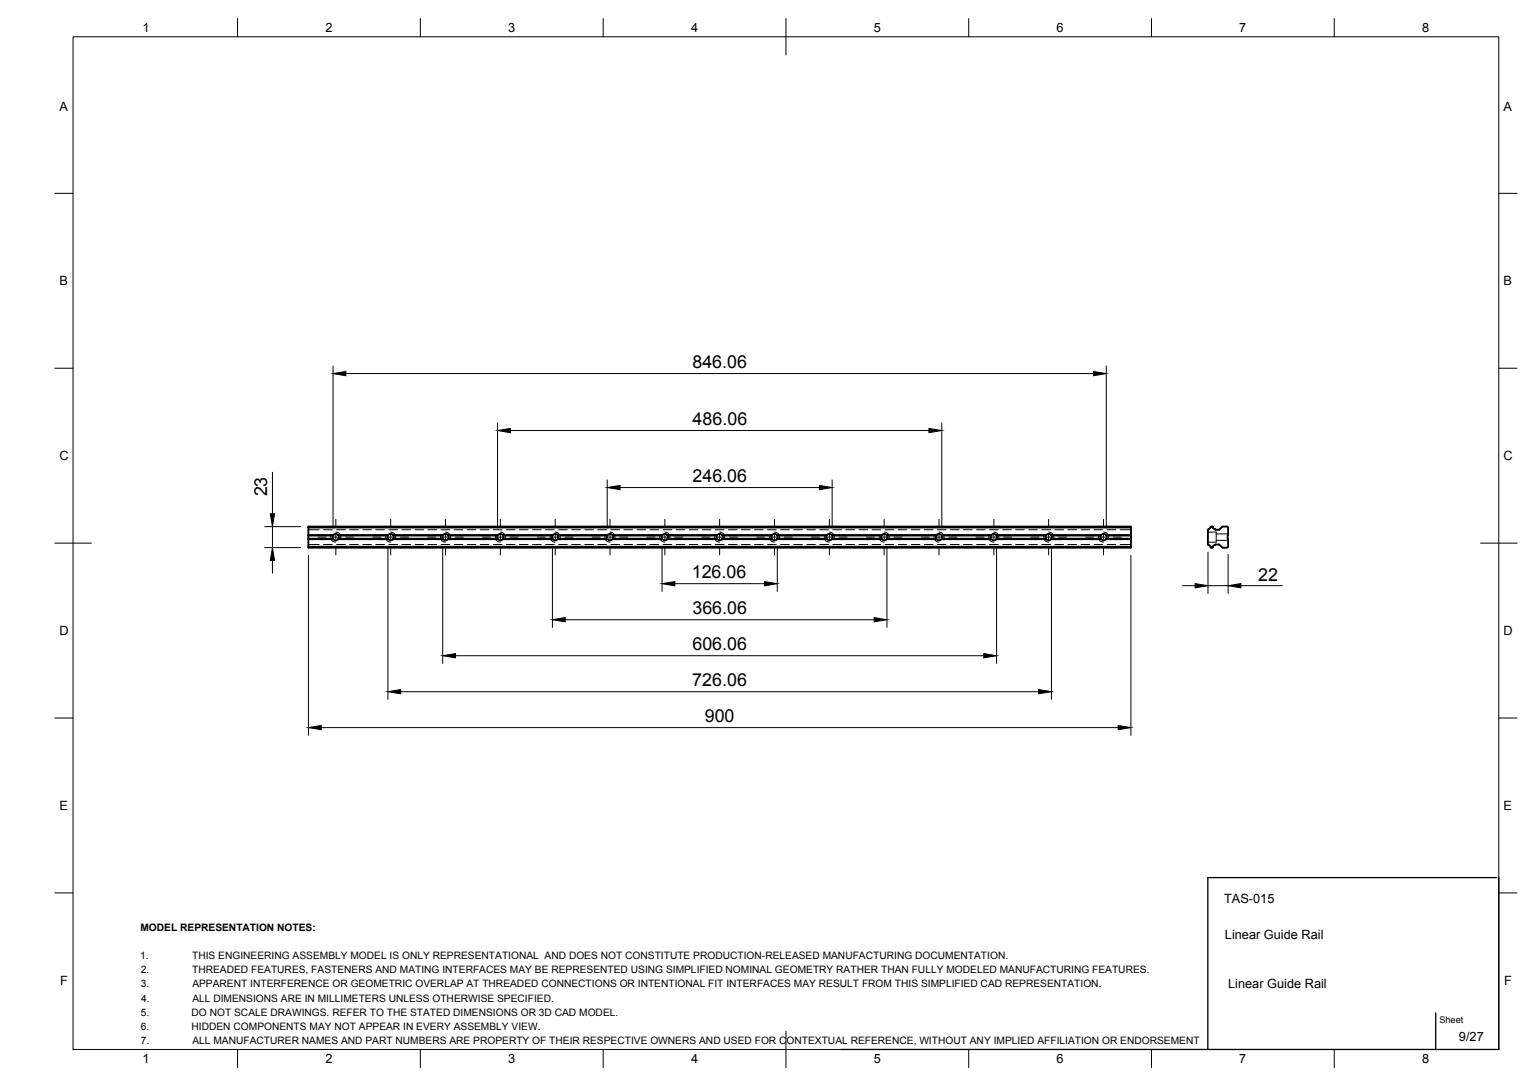
ISO-10303-21;
HEADER;
/* Generated by software containing ST-Developer
 * from STEP Tools, Inc. (www.steptools.com) 
 */

FILE_DESCRIPTION(
/* description */ ('STEP AP214'),
/* implementation_level */ '2;1');

FILE_NAME(
/* name */ 'Linear Guide Rail.step',
/* time_stamp */ '2026-11-15T14:49:54-08:00',
/* author */ (''),
/* organization */ (''),
/* preprocessor_version */ 'ST-DEVELOPER v20.2',
/* originating_system */ 'Autodesk Translation Framework v15.17.0.0',
/* authorisation */ '');

FILE_SCHEMA (('AUTOMOTIVE_DESIGN { 1 0 10303 214 3 1 1 }'));
ENDSEC;

DATA;
#10=MECHANICAL_DESIGN_GEOMETRIC_PRESENTATION_REPRESENTATION('',(#1104),#66721);
#582=ELLIPSE('',#26235,4.94974735819038,3.49999990182558);
#583=ELLIPSE('',#26237,4.94974766602105,3.5000001764392);
#584=ELLIPSE('',#26241,4.94974746762207,3.49999999945822);
#585=ELLIPSE('',#26243,4.94974743837769,3.49999997319395);
#586=ELLIPSE('',#26249,4.94974746471116,3.49999999781732);
#587=ELLIPSE('',#26251,4.94974761521235,3.50000013143823);
#588=ELLIPSE('',#26255,4.94974751536128,3.5000000426592);
#589=ELLIPSE('',#26257,4.94974734791332,3.49999989298097);
#590=ELLIPSE('',#26263,4.94974738455087,3.49999992654364);
#591=ELLIPSE('',#26265,4.94974756609828,3.50000008750549);
#592=ELLIPSE('',#26269,4.94974748465299,3.50000001559145);
#593=ELLIPSE('',#26271,4.9497474078675,3.49999994629514);
#594=ELLIPSE('',#26277,4.9497473461591,3.49999989191482);
#595=ELLIPSE('',#26279,4.94974750610666,3.50000003412937);
#596=ELLIPSE('',#26283,4.94974748783974,3.50000001743086);
#597=ELLIPSE('',#26285,4.94974744634947,3.49999998103439);
#598=ELLIPSE('',#26291,4.94974749695506,3.50000002579411);
#599=ELLIPSE('',#26293,4.94974750752024,3.50000003493957);
#600=ELLIPSE('',#26297,4.94974751315491,3.50000003982775);
#601=ELLIPSE('',#26299,4.949747463355,3.4999999955299);
#602=ELLIPSE('',#26305,4.94974749836308,3.50000002653739);
#603=ELLIPSE('',#26307,4.94974757675016,3.50000009672614);
#604=ELLIPSE('',#26311,4.94974748001691,3.50000000973653);
#605=ELLIPSE('',#26313,4.94974739716868,3.49999993702713);
#606=ELLIPSE('',#26319,4.94974749924226,3.5000000270794);
#607=ELLIPSE('',#26321,4.94974743684973,3.49999997233704);
#608=ELLIPSE('',#26325,4.9497475382208,3.50000006223073);
#609=ELLIPSE('',#26327,4.94974747235583,3.5000000037591);
#610=ELLIPSE('',#26333,4.94974748843076,3.5000000176963);
#611=ELLIPSE('',#26335,4.94974741762146,3.49999995499458);
#612=ELLIPSE('',#26339,4.94974749231943,3.50000002155544);
#613=ELLIPSE('',#26341,4.94974745849775,3.49999999105758);
#614=ELLIPSE('',#26347,4.94974743835813,3.49999997320228);
#615=ELLIPSE('',#26349,4.94974746762365,3.49999999944211);
#616=ELLIPSE('',#26353,4.94974749229401,3.50000002151707);
#617=ELLIPSE('',#26355,4.9497474430954,3.4999999775075);
#618=ELLIPSE('',#26361,4.94974746457826,3.49999999694589);
#619=ELLIPSE('',#26363,4.94974746001076,3.49999999272877);
#620=ELLIPSE('',#26367,4.94974748578252,3.50000001541321);
#621=ELLIPSE('',#26369,4.94974746533883,3.49999999735002);
#622=ELLIPSE('',#26375,4.94974749254742,3.50000002161139);
#623=ELLIPSE('',#26377,4.94974746567926,3.49999999752504);
#624=ELLIPSE('',#26381,4.94974748072687,3.50000001091353);
#625=ELLIPSE('',#26383,4.94974746232603,3.49999999483898);
#626=ELLIPSE('',#26389,4.94974748208041,3.50000001242701);
#627=ELLIPSE('',#26391,4.94974745070612,3.49999998421949);
#628=ELLIPSE('',#26395,4.94974745801903,3.49999999076925);
#629=ELLIPSE('',#26397,4.94974746302533,3.49999999523587);
#630=ELLIPSE('',#26403,4.94974746046047,3.49999999301059);
#631=ELLIPSE('',#26405,4.94974745907472,3.49999999180994);
#632=ELLIPSE('',#26409,4.94974747036828,3.50000000182558);
#633=ELLIPSE('',#26411,4.9497474701889,3.50000000171811);
#634=ELLIPSE('',#26417,4.94974746606674,3.49999999798426);
#635=ELLIPSE('',#26419,4.94974746678755,3.49999999861078);
#636=ELLIPSE('',#26423,4.94974746786117,3.49999999962962);
#637=ELLIPSE('',#26425,4.9497474685907,3.50000000019107);
#638=ELLIPSE('',#26431,4.94974746853076,3.50000000020001);
#639=ELLIPSE('',#26433,4.94974746847046,3.50000000014575);
#640=ELLIPSE('',#26437,4.9497474687332,3.50000000037123);
#641=ELLIPSE('',#26439,4.94974746865778,3.50000000030521);
#1042=SHAPE_REPRESENTATION_RELATIONSHIP('SRR','None',#66900,#1073);
#1073=ADVANCED_BREP_SHAPE_REPRESENTATION('',(#1139),#66691);
#1104=STYLED_ITEM('',(#67095),#1139);
#1139=MANIFOLD_SOLID_BREP('Body1',#25670);
#1247=FACE_BOUND('',#3970,.T.);
#1248=FACE_BOUND('',#3971,.T.);
#1249=FACE_BOUND('',#3972,.T.);
#1250=FACE_BOUND('',#3973,.T.);
#1251=FACE_BOUND('',#3974,.T.);
#1252=FACE_BOUND('',#3975,.T.);
#1253=FACE_BOUND('',#3976,.T.);
#1254=FACE_BOUND('',#3977,.T.);
#1255=FACE_BOUND('',#3978,.T.);
#1256=FACE_BOUND('',#3979,.T.);
#1257=FACE_BOUND('',#3980,.T.);
#1258=FACE_BOUND('',#3981,.T.);
#1259=FACE_BOUND('',#3982,.T.);
#1260=FACE_BOUND('',#3983,.T.);
#1261=FACE_BOUND('',#3984,.T.);
#1262=FACE_BOUND('',#4023,.T.);
#1263=FACE_BOUND('',#4025,.T.);
#1264=FACE_BOUND('',#4027,.T.);
#1265=FACE_BOUND('',#4029,.T.);
#1266=FACE_BOUND('',#4031,.T.);
#1267=FACE_BOUND('',#4033,.T.);
#1268=FACE_BOUND('',#4035,.T.);
#1269=FACE_BOUND('',#4037,.T.);
#1270=FACE_BOUND('',#4039,.T.);
#1271=FACE_BOUND('',#4041,.T.);
#1272=FACE_BOUND('',#4043,.T.);
#1273=FACE_BOUND('',#4045,.T.);
#1274=FACE_BOUND('',#4047,.T.);
#1275=FACE_BOUND('',#4049,.T.);
#1276=FACE_BOUND('',#4051,.T.);
#1551=PLANE('',#26440);
#1552=PLANE('',#26441);
#1553=PLANE('',#26442);
#1554=PLANE('',#26443);
#1555=PLANE('',#26444);
#1556=PLANE('',#26445);
#1557=PLANE('',#26446);
#1558=PLANE('',#26447);
#1559=PLANE('',#26448);
#1560=PLANE('',#26449);
#1561=PLANE('',#26450);
#1562=PLANE('',#26451);
#1563=PLANE('',#26452);
#1564=PLANE('',#26453);
#1565=PLANE('',#26454);
#1566=PLANE('',#26455);
#1567=PLANE('',#26456);
#1568=PLANE('',#26457);
#1569=PLANE('',#26458);
#1570=PLANE('',#26459);
#1571=PLANE('',#26460);
#1572=PLANE('',#26461);
#1573=PLANE('',#26462);
#1574=PLANE('',#26463);
#1575=PLANE('',#26464);
#1576=PLANE('',#26465);
#1577=PLANE('',#26466);
#1578=PLANE('',#26467);
#1579=PLANE('',#26468);
#1580=PLANE('',#26469);
#1581=PLANE('',#26470);
#1582=PLANE('',#26471);
#1583=PLANE('',#26472);
#1584=PLANE('',#26473);
#1585=PLANE('',#26474);
#1586=PLANE('',#26475);
#1587=PLANE('',#26476);
#1588=PLANE('',#26477);
#1589=PLANE('',#26478);
#1590=PLANE('',#26479);
#1591=PLANE('',#26480);
#1592=PLANE('',#26481);
#1593=PLANE('',#26482);
#1594=PLANE('',#26483);
#1595=PLANE('',#26484);
#1596=PLANE('',#26485);
#1597=PLANE('',#26486);
#1598=PLANE('',#26487);
#1599=PLANE('',#26510);
#1600=PLANE('',#26533);
#1601=PLANE('',#26534);
#1602=PLANE('',#26535);
#1603=PLANE('',#26536);
#1604=PLANE('',#26537);
#1605=PLANE('',#26538);
#1606=PLANE('',#26539);
#1607=PLANE('',#26540);
#1608=PLANE('',#26541);
#1609=PLANE('',#26542);
#1610=PLANE('',#26543);
#1611=PLANE('',#26544);
#1612=PLANE('',#26545);
#1613=PLANE('',#26546);
#1614=PLANE('',#26558);
#1615=PLANE('',#26559);
#1616=PLANE('',#26560);
#1617=PLANE('',#26561);
#1618=PLANE('',#26562);
#1619=PLANE('',#26574);
#1620=PLANE('',#26575);
#1621=PLANE('',#26576);
#1622=PLANE('',#26577);
#1623=PLANE('',#26578);
#1624=PLANE('',#26579);
#1625=PLANE('',#26580);
#1626=PLANE('',#26581);
#1627=PLANE('',#26582);
#1628=PLANE('',#26583);
#1629=PLANE('',#26584);
#1630=PLANE('',#26585);
#1631=PLANE('',#26586);
#1632=PLANE('',#26587);
#1633=PLANE('',#26588);
#1634=PLANE('',#26589);
#1635=PLANE('',#26590);
#1636=PLANE('',#26591);
#2363=FACE_OUTER_BOUND('',#3884,.T.);
#2364=FACE_OUTER_BOUND('',#3885,.T.);
#2365=FACE_OUTER_BOUND('',#3886,.T.);
#2366=FACE_OUTER_BOUND('',#3887,.T.);
#2367=FACE_OUTER_BOUND('',#3888,.T.);
#2368=FACE_OUTER_BOUND('',#3889,.T.);
#2369=FACE_OUTER_BOUND('',#3890,.T.);
#2370=FACE_OUTER_BOUND('',#3891,.T.);
#2371=FACE_OUTER_BOUND('',#3892,.T.);
#2372=FACE_OUTER_BOUND('',#3893,.T.);
#2373=FACE_OUTER_BOUND('',#3894,.T.);
#2374=FACE_OUTER_BOUND('',#3895,.T.);
#2375=FACE_OUTER_BOUND('',#3896,.T.);
#2376=FACE_OUTER_BOUND('',#3897,.T.);
#2377=FACE_OUTER_BOUND('',#3898,.T.);
#2378=FACE_OUTER_BOUND('',#3899,.T.);
#2379=FACE_OUTER_BOUND('',#3900,.T.);
#2380=FACE_OUTER_BOUND('',#3901,.T.);
#2381=FACE_OUTER_BOUND('',#3902,.T.);
#2382=FACE_OUTER_BOUND('',#3903,.T.);
#2383=FACE_OUTER_BOUND('',#3904,.T.);
#2384=FACE_OUTER_BOUND('',#3905,.T.);
#2385=FACE_OUTER_BOUND('',#3906,.T.);
#2386=FACE_OUTER_BOUND('',#3907,.T.);
#2387=FACE_OUTER_BOUND('',#3908,.T.);
#2388=FACE_OUTER_BOUND('',#3909,.T.);
#2389=FACE_OUTER_BOUND('',#3910,.T.);
#2390=FACE_OUTER_BOUND('',#3911,.T.);
#2391=FACE_OUTER_BOUND('',#3912,.T.);
#2392=FACE_OUTER_BOUND('',#3913,.T.);
#2393=FACE_OUTER_BOUND('',#3914,.T.);
#2394=FACE_OUTER_BOUND('',#3915,.T.);
#2395=FACE_OUTER_BOUND('',#3916,.T.);
#2396=FACE_OUTER_BOUND('',#3917,.T.);
#2397=FACE_OUTER_BOUND('',#3918,.T.);
#2398=FACE_OUTER_BOUND('',#3919,.T.);
#2399=FACE_OUTER_BOUND('',#3920,.T.);
#2400=FACE_OUTER_BOUND('',#3921,.T.);
#2401=FACE_OUTER_BOUND('',#3922,.T.);
#2402=FACE_OUTER_BOUND('',#3923,.T.);
#2403=FACE_OUTER_BOUND('',#3924,.T.);
#2404=FACE_OUTER_BOUND('',#3925,.T.);
#2405=FACE_OUTER_BOUND('',#3926,.T.);
#2406=FACE_OUTER_BOUND('',#3927,.T.);
#2407=FACE_OUTER_BOUND('',#3928,.T.);
#2408=FACE_OUTER_BOUND('',#3929,.T.);
#2409=FACE_OUTER_BOUND('',#3930,.T.);
#2410=FACE_OUTER_BOUND('',#3931,.T.);
#2411=FACE_OUTER_BOUND('',#3932,.T.);
#2412=FACE_OUTER_BOUND('',#3933,.T.);
#2413=FACE_OUTER_BOUND('',#3934,.T.);
#2414=FACE_OUTER_BOUND('',#3935,.T.);
#2415=FACE_OUTER_BOUND('',#3936,.T.);
#2416=FACE_OUTER_BOUND('',#3937,.T.);
#2417=FACE_OUTER_BOUND('',#3938,.T.);
#2418=FACE_OUTER_BOUND('',#3939,.T.);
#2419=FACE_OUTER_BOUND('',#3940,.T.);
#2420=FACE_OUTER_BOUND('',#3941,.T.);
#2421=FACE_OUTER_BOUND('',#3942,.T.);
#2422=FACE_OUTER_BOUND('',#3943,.T.);
#2423=FACE_OUTER_BOUND('',#3944,.T.);
#2424=FACE_OUTER_BOUND('',#3945,.T.);
#2425=FACE_OUTER_BOUND('',#3946,.T.);
#2426=FACE_OUTER_BOUND('',#3947,.T.);
#2427=FACE_OUTER_BOUND('',#3948,.T.);
#2428=FACE_OUTER_BOUND('',#3949,.T.);
#2429=FACE_OUTER_BOUND('',#3950,.T.);
#2430=FACE_OUTER_BOUND('',#3951,.T.);
#2431=FACE_OUTER_BOUND('',#3952,.T.);
#2432=FACE_OUTER_BOUND('',#3953,.T.);
#2433=FACE_OUTER_BOUND('',#3954,.T.);
#2434=FACE_OUTER_BOUND('',#3955,.T.);
#2435=FACE_OUTER_BOUND('',#3956,.T.);
#2436=FACE_OUTER_BOUND('',#3957,.T.);
#2437=FACE_OUTER_BOUND('',#3958,.T.);
#2438=FACE_OUTER_BOUND('',#3959,.T.);
#2439=FACE_OUTER_BOUND('',#3960,.T.);
#2440=FACE_OUTER_BOUND('',#3961,.T.);
#2441=FACE_OUTER_BOUND('',#3962,.T.);
#2442=FACE_OUTER_BOUND('',#3963,.T.);
#2443=FACE_OUTER_BOUND('',#3964,.T.);
#2444=FACE_OUTER_BOUND('',#3965,.T.);
#2445=FACE_OUTER_BOUND('',#3966,.T.);
#2446=FACE_OUTER_BOUND('',#3967,.T.);
#2447=FACE_OUTER_BOUND('',#3968,.T.);
#2448=FACE_OUTER_BOUND('',#3969,.T.);
#2449=FACE_OUTER_BOUND('',#3985,.T.);
#2450=FACE_OUTER_BOUND('',#3986,.T.);
#2451=FACE_OUTER_BOUND('',#3987,.T.);
#2452=FACE_OUTER_BOUND('',#3988,.T.);
#2453=FACE_OUTER_BOUND('',#3989,.T.);
#2454=FACE_OUTER_BOUND('',#3990,.T.);
#2455=FACE_OUTER_BOUND('',#3991,.T.);
#2456=FACE_OUTER_BOUND('',#3992,.T.);
#2457=FACE_OUTER_BOUND('',#3993,.T.);
#2458=FACE_OUTER_BOUND('',#3994,.T.);
#2459=FACE_OUTER_BOUND('',#3995,.T.);
#2460=FACE_OUTER_BOUND('',#3996,.T.);
#2461=FACE_OUTER_BOUND('',#3997,.T.);
#2462=FACE_OUTER_BOUND('',#3998,.T.);
#2463=FACE_OUTER_BOUND('',#3999,.T.);
#2464=FACE_OUTER_BOUND('',#4000,.T.);
#2465=FACE_OUTER_BOUND('',#4001,.T.);
#2466=FACE_OUTER_BOUND('',#4002,.T.);
#2467=FACE_OUTER_BOUND('',#4003,.T.);
#2468=FACE_OUTER_BOUND('',#4004,.T.);
#2469=FACE_OUTER_BOUND('',#4005,.T.);
#2470=FACE_OUTER_BOUND('',#4006,.T.);
#2471=FACE_OUTER_BOUND('',#4007,.T.);
#2472=FACE_OUTER_BOUND('',#4008,.T.);
#2473=FACE_OUTER_BOUND('',#4009,.T.);
#2474=FACE_OUTER_BOUND('',#4010,.T.);
#2475=FACE_OUTER_BOUND('',#4011,.T.);
#2476=FACE_OUTER_BOUND('',#4012,.T.);
#2477=FACE_OUTER_BOUND('',#4013,.T.);
#2478=FACE_OUTER_BOUND('',#4014,.T.);
#2479=FACE_OUTER_BOUND('',#4015,.T.);
#2480=FACE_OUTER_BOUND('',#4016,.T.);
#2481=FACE_OUTER_BOUND('',#4017,.T.);
#2482=FACE_OUTER_BOUND('',#4018,.T.);
#2483=FACE_OUTER_BOUND('',#4019,.T.);
#2484=FACE_OUTER_BOUND('',#4020,.T.);
#2485=FACE_OUTER_BOUND('',#4021,.T.);
#2486=FACE_OUTER_BOUND('',#4022,.T.);
#2487=FACE_OUTER_BOUND('',#4024,.T.);
#2488=FACE_OUTER_BOUND('',#4026,.T.);
#2489=FACE_OUTER_BOUND('',#4028,.T.);
#2490=FACE_OUTER_BOUND('',#4030,.T.);
#2491=FACE_OUTER_BOUND('',#4032,.T.);
#2492=FACE_OUTER_BOUND('',#4034,.T.);
#2493=FACE_OUTER_BOUND('',#4036,.T.);
#2494=FACE_OUTER_BOUND('',#4038,.T.);
#2495=FACE_OUTER_BOUND('',#4040,.T.);
#2496=FACE_OUTER_BOUND('',#4042,.T.);
#2497=FACE_OUTER_BOUND('',#4044,.T.);
#2498=FACE_OUTER_BOUND('',#4046,.T.);
#2499=FACE_OUTER_BOUND('',#4048,.T.);
#2500=FACE_OUTER_BOUND('',#4050,.T.);
#3884=EDGE_LOOP('',(#17068,#17069,#17070,#17071));
#3885=EDGE_LOOP('',(#17072,#17073,#17074,#17075,#17076,#17077,#17078,#17079,
#17080,#17081,#17082,#17083));
#3886=EDGE_LOOP('',(#17084,#17085,#17086,#17087));
#3887=EDGE_LOOP('',(#17088,#17089,#17090,#17091,#17092,#17093,#17094,#17095,
#17096,#17097,#17098,#17099));
#3888=EDGE_LOOP('',(#17100,#17101,#17102,#17103));
#3889=EDGE_LOOP('',(#17104,#17105,#17106,#17107,#17108,#17109,#17110,#17111,
#17112,#17113,#17114,#17115));
#3890=EDGE_LOOP('',(#17116,#17117,#17118,#17119));
#3891=EDGE_LOOP('',(#17120,#17121,#17122,#17123,#17124,#17125,#17126,#17127,
#17128,#17129,#17130,#17131));
#3892=EDGE_LOOP('',(#17132,#17133,#17134,#17135));
#3893=EDGE_LOOP('',(#17136,#17137,#17138,#17139,#17140,#17141,#17142,#17143,
#17144,#17145,#17146,#17147));
#3894=EDGE_LOOP('',(#17148,#17149,#17150,#17151));
#3895=EDGE_LOOP('',(#17152,#17153,#17154,#17155,#17156,#17157,#17158,#17159,
#17160,#17161,#17162,#17163));
#3896=EDGE_LOOP('',(#17164,#17165,#17166,#17167));
#3897=EDGE_LOOP('',(#17168,#17169,#17170,#17171,#17172,#17173,#17174,#17175,
#17176,#17177,#17178,#17179));
#3898=EDGE_LOOP('',(#17180,#17181,#17182,#17183));
#3899=EDGE_LOOP('',(#17184,#17185,#17186,#17187,#17188,#17189,#17190,#17191,
#17192,#17193,#17194,#17195));
#3900=EDGE_LOOP('',(#17196,#17197,#17198,#17199));
#3901=EDGE_LOOP('',(#17200,#17201,#17202,#17203,#17204,#17205,#17206,#17207,
#17208,#17209,#17210,#17211));
#3902=EDGE_LOOP('',(#17212,#17213,#17214,#17215));
#3903=EDGE_LOOP('',(#17216,#17217,#17218,#17219,#17220,#17221,#17222,#17223,
#17224,#17225,#17226,#17227));
#3904=EDGE_LOOP('',(#17228,#17229,#17230,#17231));
#3905=EDGE_LOOP('',(#17232,#17233,#17234,#17235,#17236,#17237,#17238,#17239,
#17240,#17241,#17242,#17243));
#3906=EDGE_LOOP('',(#17244,#17245,#17246,#17247));
#3907=EDGE_LOOP('',(#17248,#17249,#17250,#17251,#17252,#17253,#17254,#17255,
#17256,#17257,#17258,#17259));
#3908=EDGE_LOOP('',(#17260,#17261,#17262,#17263));
#3909=EDGE_LOOP('',(#17264,#17265,#17266,#17267,#17268,#17269,#17270,#17271,
#17272,#17273,#17274,#17275));
#3910=EDGE_LOOP('',(#17276,#17277,#17278,#17279));
#3911=EDGE_LOOP('',(#17280,#17281,#17282,#17283,#17284,#17285,#17286,#17287,
#17288,#17289,#17290,#17291));
#3912=EDGE_LOOP('',(#17292,#17293,#17294,#17295));
#3913=EDGE_LOOP('',(#17296,#17297,#17298,#17299,#17300,#17301,#17302,#17303,
#17304,#17305,#17306,#17307));
#3914=EDGE_LOOP('',(#17308,#17309,#17310,#17311));
#3915=EDGE_LOOP('',(#17312,#17313,#17314,#17315));
#3916=EDGE_LOOP('',(#17316,#17317,#17318,#17319,#17320,#17321,#17322,#17323,
#17324,#17325,#17326,#17327,#17328,#17329,#17330,#17331,#17332,#17333,#17334,
#17335,#17336,#17337,#17338,#17339,#17340,#17341,#17342,#17343,#17344,#17345,
#17346,#17347,#17348,#17349));
#3917=EDGE_LOOP('',(#17350,#17351,#17352,#17353,#17354));
#3918=EDGE_LOOP('',(#17355,#17356,#17357,#17358,#17359,#17360,#17361,#17362,
#17363,#17364,#17365,#17366,#17367,#17368,#17369,#17370,#17371,#17372,#17373,
#17374,#17375,#17376,#17377,#17378,#17379,#17380,#17381,#17382,#17383,#17384,
#17385,#17386,#17387,#17388));
#3919=EDGE_LOOP('',(#17389,#17390,#17391,#17392));
#3920=EDGE_LOOP('',(#17393,#17394,#17395,#17396,#17397));
#3921=EDGE_LOOP('',(#17398,#17399,#17400,#17401));
#3922=EDGE_LOOP('',(#17402,#17403,#17404,#17405));
#3923=EDGE_LOOP('',(#17406,#17407,#17408,#17409,#17410));
#3924=EDGE_LOOP('',(#17411,#17412,#17413,#17414));
#3925=EDGE_LOOP('',(#17415,#17416,#17417,#17418));
#3926=EDGE_LOOP('',(#17419,#17420,#17421,#17422,#17423));
#3927=EDGE_LOOP('',(#17424,#17425,#17426,#17427));
#3928=EDGE_LOOP('',(#17428,#17429,#17430,#17431));
#3929=EDGE_LOOP('',(#17432,#17433,#17434,#17435,#17436));
#3930=EDGE_LOOP('',(#17437,#17438,#17439,#17440));
#3931=EDGE_LOOP('',(#17441,#17442,#17443,#17444));
#3932=EDGE_LOOP('',(#17445,#17446,#17447,#17448,#17449));
#3933=EDGE_LOOP('',(#17450,#17451,#17452,#17453));
#3934=EDGE_LOOP('',(#17454,#17455,#17456,#17457));
#3935=EDGE_LOOP('',(#17458,#17459,#17460,#17461,#17462));
#3936=EDGE_LOOP('',(#17463,#17464,#17465,#17466));
#3937=EDGE_LOOP('',(#17467,#17468,#17469,#17470));
#3938=EDGE_LOOP('',(#17471,#17472,#17473,#17474,#17475));
#3939=EDGE_LOOP('',(#17476,#17477,#17478,#17479));
#3940=EDGE_LOOP('',(#17480,#17481,#17482,#17483));
#3941=EDGE_LOOP('',(#17484,#17485,#17486,#17487,#17488));
#3942=EDGE_LOOP('',(#17489,#17490,#17491,#17492));
#3943=EDGE_LOOP('',(#17493,#17494,#17495,#17496));
#3944=EDGE_LOOP('',(#17497,#17498,#17499,#17500,#17501));
#3945=EDGE_LOOP('',(#17502,#17503,#17504,#17505));
#3946=EDGE_LOOP('',(#17506,#17507,#17508,#17509,#17510));
#3947=EDGE_LOOP('',(#17511,#17512,#17513,#17514));
#3948=EDGE_LOOP('',(#17515,#17516,#17517,#17518));
#3949=EDGE_LOOP('',(#17519,#17520,#17521,#17522));
#3950=EDGE_LOOP('',(#17523,#17524,#17525,#17526,#17527));
#3951=EDGE_LOOP('',(#17528,#17529,#17530,#17531));
#3952=EDGE_LOOP('',(#17532,#17533,#17534,#17535));
#3953=EDGE_LOOP('',(#17536,#17537,#17538,#17539,#17540));
#3954=EDGE_LOOP('',(#17541,#17542,#17543,#17544));
#3955=EDGE_LOOP('',(#17545,#17546,#17547,#17548,#17549));
#3956=EDGE_LOOP('',(#17550,#17551,#17552,#17553));
#3957=EDGE_LOOP('',(#17554,#17555,#17556,#17557));
#3958=EDGE_LOOP('',(#17558,#17559,#17560,#17561));
#3959=EDGE_LOOP('',(#17562,#17563,#17564,#17565));
#3960=EDGE_LOOP('',(#17566,#17567,#17568,#17569));
#3961=EDGE_LOOP('',(#17570,#17571,#17572,#17573,#17574,#17575,#17576,#17577,
#17578,#17579,#17580,#17581,#17582,#17583,#17584,#17585,#17586,#17587,#17588,
#17589,#17590,#17591,#17592,#17593,#17594,#17595,#17596,#17597,#17598,#17599,
#17600,#17601,#17602,#17603,#17604,#17605,#17606,#17607,#17608,#17609,#17610,
#17611,#17612,#17613,#17614,#17615));
#3962=EDGE_LOOP('',(#17616,#17617,#17618,#17619,#17620,#17621,#17622,#17623,
#17624,#17625,#17626,#17627,#17628,#17629,#17630,#17631,#17632,#17633,#17634,
#17635,#17636,#17637,#17638,#17639,#17640,#17641,#17642,#17643,#17644,#17645,
#17646,#17647,#17648,#17649,#17650,#17651,#17652,#17653,#17654,#17655,#17656,
#17657,#17658,#17659,#17660,#17661));
#3963=EDGE_LOOP('',(#17662,#17663,#17664,#17665));
#3964=EDGE_LOOP('',(#17666,#17667,#17668,#17669));
#3965=EDGE_LOOP('',(#17670,#17671,#17672,#17673));
#3966=EDGE_LOOP('',(#17674,#17675,#17676,#17677));
#3967=EDGE_LOOP('',(#17678,#17679,#17680,#17681));
#3968=EDGE_LOOP('',(#17682,#17683,#17684,#17685));
#3969=EDGE_LOOP('',(#17686,#17687,#17688,#17689));
#3970=EDGE_LOOP('',(#17690));
#3971=EDGE_LOOP('',(#17691));
#3972=EDGE_LOOP('',(#17692));
#3973=EDGE_LOOP('',(#17693));
#3974=EDGE_LOOP('',(#17694));
#3975=EDGE_LOOP('',(#17695));
#3976=EDGE_LOOP('',(#17696));
#3977=EDGE_LOOP('',(#17697));
#3978=EDGE_LOOP('',(#17698));
#3979=EDGE_LOOP('',(#17699));
#3980=EDGE_LOOP('',(#17700));
#3981=EDGE_LOOP('',(#17701));
#3982=EDGE_LOOP('',(#17702));
#3983=EDGE_LOOP('',(#17703));
#3984=EDGE_LOOP('',(#17704));
#3985=EDGE_LOOP('',(#17705,#17706,#17707,#17708));
#3986=EDGE_LOOP('',(#17709,#17710,#17711,#17712));
#3987=EDGE_LOOP('',(#17713,#17714,#17715,#17716));
#3988=EDGE_LOOP('',(#17717,#17718,#17719,#17720));
#3989=EDGE_LOOP('',(#17721,#17722,#17723,#17724));
#3990=EDGE_LOOP('',(#17725,#17726,#17727,#17728));
#3991=EDGE_LOOP('',(#17729,#17730,#17731,#17732));
#3992=EDGE_LOOP('',(#17733,#17734,#17735,#17736));
#3993=EDGE_LOOP('',(#17737,#17738,#17739,#17740));
#3994=EDGE_LOOP('',(#17741,#17742,#17743,#17744));
#3995=EDGE_LOOP('',(#17745,#17746,#17747,#17748));
#3996=EDGE_LOOP('',(#17749,#17750,#17751,#17752));
#3997=EDGE_LOOP('',(#17753,#17754,#17755,#17756));
#3998=EDGE_LOOP('',(#17757,#17758,#17759,#17760));
#3999=EDGE_LOOP('',(#17761,#17762,#17763,#17764));
#4000=EDGE_LOOP('',(#17765,#17766,#17767,#17768));
#4001=EDGE_LOOP('',(#17769,#17770,#17771,#17772));
#4002=EDGE_LOOP('',(#17773,#17774,#17775,#17776));
#4003=EDGE_LOOP('',(#17777,#17778,#17779,#17780));
#4004=EDGE_LOOP('',(#17781,#17782,#17783,#17784));
#4005=EDGE_LOOP('',(#17785,#17786,#17787,#17788));
#4006=EDGE_LOOP('',(#17789,#17790,#17791,#17792));
#4007=EDGE_LOOP('',(#17793,#17794,#17795,#17796));
#4008=EDGE_LOOP('',(#17797,#17798,#17799,#17800));
#4009=EDGE_LOOP('',(#17801,#17802,#17803,#17804));
#4010=EDGE_LOOP('',(#17805,#17806,#17807,#17808));
#4011=EDGE_LOOP('',(#17809,#17810,#17811,#17812));
#4012=EDGE_LOOP('',(#17813,#17814,#17815,#17816));
#4013=EDGE_LOOP('',(#17817,#17818,#17819,#17820));
#4014=EDGE_LOOP('',(#17821,#17822,#17823,#17824));
#4015=EDGE_LOOP('',(#17825,#17826,#17827,#17828));
#4016=EDGE_LOOP('',(#17829,#17830,#17831,#17832));
#4017=EDGE_LOOP('',(#17833,#17834,#17835,#17836));
#4018=EDGE_LOOP('',(#17837,#17838,#17839,#17840));
#4019=EDGE_LOOP('',(#17841,#17842,#17843,#17844));
#4020=EDGE_LOOP('',(#17845,#17846,#17847,#17848,#17849));
#4021=EDGE_LOOP('',(#17850,#17851,#17852,#17853));
#4022=EDGE_LOOP('',(#17854));
#4023=EDGE_LOOP('',(#17855));
#4024=EDGE_LOOP('',(#17856));
#4025=EDGE_LOOP('',(#17857));
#4026=EDGE_LOOP('',(#17858));
#4027=EDGE_LOOP('',(#17859));
#4028=EDGE_LOOP('',(#17860));
#4029=EDGE_LOOP('',(#17861));
#4030=EDGE_LOOP('',(#17862));
#4031=EDGE_LOOP('',(#17863));
#4032=EDGE_LOOP('',(#17864));
#4033=EDGE_LOOP('',(#17865));
#4034=EDGE_LOOP('',(#17866));
#4035=EDGE_LOOP('',(#17867));
#4036=EDGE_LOOP('',(#17868));
#4037=EDGE_LOOP('',(#17869));
#4038=EDGE_LOOP('',(#17870));
#4039=EDGE_LOOP('',(#17871));
#4040=EDGE_LOOP('',(#17872));
#4041=EDGE_LOOP('',(#17873));
#4042=EDGE_LOOP('',(#17874));
#4043=EDGE_LOOP('',(#17875));
#4044=EDGE_LOOP('',(#17876));
#4045=EDGE_LOOP('',(#17877));
#4046=EDGE_LOOP('',(#17878));
#4047=EDGE_LOOP('',(#17879));
#4048=EDGE_LOOP('',(#17880));
#4049=EDGE_LOOP('',(#17881));
#4050=EDGE_LOOP('',(#17882));
#4051=EDGE_LOOP('',(#17883));
#5638=LINE('',#36681,#7627);
#5639=LINE('',#36696,#7628);
#5640=LINE('',#36709,#7629);
#5641=LINE('',#36724,#7630);
#5642=LINE('',#36737,#7631);
#5643=LINE('',#36752,#7632);
#5644=LINE('',#36765,#7633);
#5645=LINE('',#36780,#7634);
#5646=LINE('',#36793,#7635);
#5647=LINE('',#36808,#7636);
#5648=LINE('',#36821,#7637);
#5649=LINE('',#36836,#7638);
#5650=LINE('',#36849,#7639);
#5651=LINE('',#36864,#7640);
#5652=LINE('',#36877,#7641);
#5653=LINE('',#36892,#7642);
#5654=LINE('',#36905,#7643);
#5655=LINE('',#36920,#7644);
#5656=LINE('',#36933,#7645);
#5657=LINE('',#36948,#7646);
#5658=LINE('',#36961,#7647);
#5659=LINE('',#36976,#7648);
#5660=LINE('',#36989,#7649);
#5661=LINE('',#37004,#7650);
#5662=LINE('',#37017,#7651);
#5663=LINE('',#37032,#7652);
#5664=LINE('',#37045,#7653);
#5665=LINE('',#37060,#7654);
#5666=LINE('',#37073,#7655);
#5667=LINE('',#37088,#7656);
#5668=LINE('',#37099,#7657);
#5669=LINE('',#37101,#7658);
#5670=LINE('',#37102,#7659);
#5671=LINE('',#37104,#7660);
#5672=LINE('',#37105,#7661);
#5673=LINE('',#37107,#7662);
#5674=LINE('',#37108,#7663);
#5675=LINE('',#37109,#7664);
#5676=LINE('',#37110,#7665);
#5677=LINE('',#37111,#7666);
#5678=LINE('',#37112,#7667);
#5679=LINE('',#37113,#7668);
#5680=LINE('',#37114,#7669);
#5681=LINE('',#37115,#7670);
#5682=LINE('',#37116,#7671);
#5683=LINE('',#37117,#7672);
#5684=LINE('',#37118,#7673);
#5685=LINE('',#37119,#7674);
#5686=LINE('',#37120,#7675);
#5687=LINE('',#37122,#7676);
#5688=LINE('',#37124,#7677);
#5689=LINE('',#37126,#7678);
#5690=LINE('',#37127,#7679);
#5691=LINE('',#37129,#7680);
#5692=LINE('',#37132,#7681);
#5693=LINE('',#37134,#7682);
#5694=LINE('',#37136,#7683);
#5695=LINE('',#37138,#7684);
#5696=LINE('',#37139,#7685);
#5697=LINE('',#37140,#7686);
#5698=LINE('',#37141,#7687);
#5699=LINE('',#37142,#7688);
#5700=LINE('',#37143,#7689);
#5701=LINE('',#37144,#7690);
#5702=LINE('',#37145,#7691);
#5703=LINE('',#37146,#7692);
#5704=LINE('',#37147,#7693);
#5705=LINE('',#37148,#7694);
#5706=LINE('',#37149,#7695);
#5707=LINE('',#37150,#7696);
#5708=LINE('',#37151,#7697);
#5709=LINE('',#37152,#7698);
#5710=LINE('',#37155,#7699);
#5711=LINE('',#37156,#7700);
#5712=LINE('',#37160,#7701);
#5713=LINE('',#37161,#7702);
#5714=LINE('',#37165,#7703);
#5715=LINE('',#37166,#7704);
#5716=LINE('',#37170,#7705);
#5717=LINE('',#37171,#7706);
#5718=LINE('',#37175,#7707);
#5719=LINE('',#37176,#7708);
#5720=LINE('',#37180,#7709);
#5721=LINE('',#37181,#7710);
#5722=LINE('',#37185,#7711);
#5723=LINE('',#37186,#7712);
#5724=LINE('',#37190,#7713);
#5725=LINE('',#37191,#7714);
#5726=LINE('',#37195,#7715);
#5727=LINE('',#37196,#7716);
#5728=LINE('',#37199,#7717);
#5729=LINE('',#37200,#7718);
#5730=LINE('',#37205,#7719);
#5731=LINE('',#37206,#7720);
#5732=LINE('',#37210,#7721);
#5733=LINE('',#37211,#7722);
#5734=LINE('',#37214,#7723);
#5735=LINE('',#37215,#7724);
#5736=LINE('',#37220,#7725);
#5737=LINE('',#37222,#7726);
#5738=LINE('',#37223,#7727);
#5739=LINE('',#37226,#7728);
#5740=LINE('',#37229,#7729);
#5741=LINE('',#37231,#7730);
#5742=LINE('',#37235,#7731);
#5743=LINE('',#37239,#7732);
#5744=LINE('',#37243,#7733);
#5745=LINE('',#37251,#7734);
#5746=LINE('',#37255,#7735);
#5747=LINE('',#37259,#7736);
#5748=LINE('',#37267,#7737);
#5749=LINE('',#37269,#7738);
#5750=LINE('',#37271,#7739);
#5751=LINE('',#37279,#7740);
#5752=LINE('',#37283,#7741);
#5753=LINE('',#37287,#7742);
#5754=LINE('',#37295,#7743);
#5755=LINE('',#37299,#7744);
#5756=LINE('',#37303,#7745);
#5757=LINE('',#37307,#7746);
#5758=LINE('',#37308,#7747);
#5759=LINE('',#37310,#7748);
#5760=LINE('',#37311,#7749);
#5761=LINE('',#37313,#7750);
#5762=LINE('',#37315,#7751);
#5763=LINE('',#37317,#7752);
#5764=LINE('',#37321,#7753);
#5765=LINE('',#37325,#7754);
#5766=LINE('',#37329,#7755);
#5767=LINE('',#37337,#7756);
#5768=LINE('',#37341,#7757);
#5769=LINE('',#37345,#7758);
#5770=LINE('',#37353,#7759);
#5771=LINE('',#37355,#7760);
#5772=LINE('',#37357,#7761);
#5773=LINE('',#37365,#7762);
#5774=LINE('',#37369,#7763);
#5775=LINE('',#37373,#7764);
#5776=LINE('',#37381,#7765);
#5777=LINE('',#37385,#7766);
#5778=LINE('',#37389,#7767);
#5779=LINE('',#37393,#7768);
#5780=LINE('',#37394,#7769);
#5781=LINE('',#37396,#7770);
#5782=LINE('',#37397,#7771);
#5783=LINE('',#37399,#7772);
#5784=LINE('',#37400,#7773);
#5785=LINE('',#37402,#7774);
#5786=LINE('',#37403,#7775);
#5787=LINE('',#37405,#7776);
#5788=LINE('',#37406,#7777);
#5789=LINE('',#37408,#7778);
#5790=LINE('',#37409,#7779);
#5791=LINE('',#37411,#7780);
#5792=LINE('',#37412,#7781);
#5793=LINE('',#37414,#7782);
#5794=LINE('',#37416,#7783);
#5795=LINE('',#37418,#7784);
#5796=LINE('',#37420,#7785);
#5797=LINE('',#37421,#7786);
#5798=LINE('',#37423,#7787);
#5799=LINE('',#37424,#7788);
#5800=LINE('',#37426,#7789);
#5801=LINE('',#37427,#7790);
#5802=LINE('',#37429,#7791);
#5803=LINE('',#37430,#7792);
#5804=LINE('',#37432,#7793);
#5805=LINE('',#37434,#7794);
#5806=LINE('',#37435,#7795);
#5807=LINE('',#37437,#7796);
#5808=LINE('',#37438,#7797);
#5809=LINE('',#37449,#7798);
#5810=LINE('',#37450,#7799);
#5811=LINE('',#37452,#7800);
#5812=LINE('',#37453,#7801);
#5813=LINE('',#37455,#7802);
#5814=LINE('',#37456,#7803);
#5815=LINE('',#37458,#7804);
#5816=LINE('',#37459,#7805);
#5817=LINE('',#37462,#7806);
#5818=LINE('',#37463,#7807);
#5819=LINE('',#37465,#7808);
#5820=LINE('',#37466,#7809);
#5821=LINE('',#37478,#7810);
#7627=VECTOR('',#29293,5.49999999999995);
#7628=VECTOR('',#29308,3.49999999999995);
#7629=VECTOR('',#29323,5.49999999999995);
#7630=VECTOR('',#29338,3.49999999999995);
#7631=VECTOR('',#29353,5.49999999999995);
#7632=VECTOR('',#29368,3.49999999999995);
#7633=VECTOR('',#29383,5.49999999999995);
#7634=VECTOR('',#29398,3.49999999999995);
#7635=VECTOR('',#29413,5.49999999999995);
#7636=VECTOR('',#29428,3.49999999999995);
#7637=VECTOR('',#29443,5.49999999999995);
#7638=VECTOR('',#29458,3.49999999999995);
#7639=VECTOR('',#29473,5.50000000000001);
#7640=VECTOR('',#29488,3.5);
#7641=VECTOR('',#29503,5.50000000000001);
#7642=VECTOR('',#29518,3.5);
#7643=VECTOR('',#29533,5.50000000000001);
#7644=VECTOR('',#29548,3.5);
#7645=VECTOR('',#29563,5.50000000000001);
#7646=VECTOR('',#29578,3.5);
#7647=VECTOR('',#29593,5.50000000000001);
#7648=VECTOR('',#29608,3.5);
#7649=VECTOR('',#29623,5.50000000000001);
#7650=VECTOR('',#29638,3.5);
#7651=VECTOR('',#29653,5.50000000000001);
#7652=VECTOR('',#29668,3.5);
#7653=VECTOR('',#29683,5.5);
#7654=VECTOR('',#29698,3.5);
#7655=VECTOR('',#29713,5.5);
#7656=VECTOR('',#29728,3.5);
#7657=VECTOR('',#29741,1000.);
#7658=VECTOR('',#29742,1000.);
#7659=VECTOR('',#29743,1000.);
#7660=VECTOR('',#29746,1000.);
#7661=VECTOR('',#29747,1000.);
#7662=VECTOR('',#29750,1000.);
#7663=VECTOR('',#29751,1000.);
#7664=VECTOR('',#29752,1000.);
#7665=VECTOR('',#29753,1000.);
#7666=VECTOR('',#29754,1000.);
#7667=VECTOR('',#29755,1000.);
#7668=VECTOR('',#29756,1000.);
#7669=VECTOR('',#29757,1000.);
#7670=VECTOR('',#29758,1000.);
#7671=VECTOR('',#29759,1000.);
#7672=VECTOR('',#29760,1000.);
#7673=VECTOR('',#29761,1000.);
#7674=VECTOR('',#29762,1000.);
#7675=VECTOR('',#29763,1000.);
#7676=VECTOR('',#29764,1000.);
#7677=VECTOR('',#29765,1000.);
#7678=VECTOR('',#29766,1000.);
#7679=VECTOR('',#29767,1000.);
#7680=VECTOR('',#29770,1000.);
#7681=VECTOR('',#29773,1000.);
#7682=VECTOR('',#29774,1000.);
#7683=VECTOR('',#29775,1000.);
#7684=VECTOR('',#29776,1000.);
#7685=VECTOR('',#29777,1000.);
#7686=VECTOR('',#29778,1000.);
#7687=VECTOR('',#29779,1000.);
#7688=VECTOR('',#29780,1000.);
#7689=VECTOR('',#29781,1000.);
#7690=VECTOR('',#29782,1000.);
#7691=VECTOR('',#29783,1000.);
#7692=VECTOR('',#29784,1000.);
#7693=VECTOR('',#29785,1000.);
#7694=VECTOR('',#29786,1000.);
#7695=VECTOR('',#29787,1000.);
#7696=VECTOR('',#29788,1000.);
#7697=VECTOR('',#29789,1000.);
#7698=VECTOR('',#29790,1000.);
#7699=VECTOR('',#29795,1000.);
#7700=VECTOR('',#29796,1000.);
#7701=VECTOR('',#29803,1000.);
#7702=VECTOR('',#29804,1000.);
#7703=VECTOR('',#29811,1000.);
#7704=VECTOR('',#29812,1000.);
#7705=VECTOR('',#29819,1000.);
#7706=VECTOR('',#29820,1000.);
#7707=VECTOR('',#29827,1000.);
#7708=VECTOR('',#29828,1000.);
#7709=VECTOR('',#29835,1000.);
#7710=VECTOR('',#29836,1000.);
#7711=VECTOR('',#29843,1000.);
#7712=VECTOR('',#29844,1000.);
#7713=VECTOR('',#29851,1000.);
#7714=VECTOR('',#29852,1000.);
#7715=VECTOR('',#29859,1000.);
#7716=VECTOR('',#29860,1000.);
#7717=VECTOR('',#29865,1000.);
#7718=VECTOR('',#29866,1000.);
#7719=VECTOR('',#29875,1000.);
#7720=VECTOR('',#29876,1000.);
#7721=VECTOR('',#29883,1000.);
#7722=VECTOR('',#29884,1000.);
#7723=VECTOR('',#29889,1000.);
#7724=VECTOR('',#29890,1000.);
#7725=VECTOR('',#29897,1000.);
#7726=VECTOR('',#29898,1000.);
#7727=VECTOR('',#29899,1000.);
#7728=VECTOR('',#29904,1000.);
#7729=VECTOR('',#29907,1000.);
#7730=VECTOR('',#29908,1000.);
#7731=VECTOR('',#29911,1000.);
#7732=VECTOR('',#29914,1000.);
#7733=VECTOR('',#29917,1000.);
#7734=VECTOR('',#29924,1000.);
#7735=VECTOR('',#29927,1000.);
#7736=VECTOR('',#29930,1000.);
#7737=VECTOR('',#29937,1000.);
#7738=VECTOR('',#29938,1000.);
#7739=VECTOR('',#29939,1000.);
#7740=VECTOR('',#29946,1000.);
#7741=VECTOR('',#29949,1000.);
#7742=VECTOR('',#29952,1000.);
#7743=VECTOR('',#29959,1000.);
#7744=VECTOR('',#29962,1000.);
#7745=VECTOR('',#29965,1000.);
#7746=VECTOR('',#29968,1000.);
#7747=VECTOR('',#29969,1000.);
#7748=VECTOR('',#29970,1000.);
#7749=VECTOR('',#29971,1000.);
#7750=VECTOR('',#29974,1000.);
#7751=VECTOR('',#29975,1000.);
#7752=VECTOR('',#29976,1000.);
#7753=VECTOR('',#29979,1000.);
#7754=VECTOR('',#29982,1000.);
#7755=VECTOR('',#29985,1000.);
#7756=VECTOR('',#29992,1000.);
#7757=VECTOR('',#29995,1000.);
#7758=VECTOR('',#29998,1000.);
#7759=VECTOR('',#30005,1000.);
#7760=VECTOR('',#30006,1000.);
#7761=VECTOR('',#30007,1000.);
#7762=VECTOR('',#30014,1000.);
#7763=VECTOR('',#30017,1000.);
#7764=VECTOR('',#30020,1000.);
#7765=VECTOR('',#30027,1000.);
#7766=VECTOR('',#30030,1000.);
#7767=VECTOR('',#30033,1000.);
#7768=VECTOR('',#30036,1000.);
#7769=VECTOR('',#30037,1000.);
#7770=VECTOR('',#30040,1000.);
#7771=VECTOR('',#30041,1000.);
#7772=VECTOR('',#30044,1000.);
#7773=VECTOR('',#30045,1000.);
#7774=VECTOR('',#30048,1000.);
#7775=VECTOR('',#30049,1000.);
#7776=VECTOR('',#30052,1000.);
#7777=VECTOR('',#30053,1000.);
#7778=VECTOR('',#30056,1000.);
#7779=VECTOR('',#30057,1000.);
#7780=VECTOR('',#30060,1000.);
#7781=VECTOR('',#30061,1000.);
#7782=VECTOR('',#30064,1000.);
#7783=VECTOR('',#30067,1000.);
#7784=VECTOR('',#30070,1000.);
#7785=VECTOR('',#30073,1000.);
#7786=VECTOR('',#30074,1000.);
#7787=VECTOR('',#30077,1000.);
#7788=VECTOR('',#30078,1000.);
#7789=VECTOR('',#30081,1000.);
#7790=VECTOR('',#30082,1000.);
#7791=VECTOR('',#30085,1000.);
#7792=VECTOR('',#30086,1000.);
#7793=VECTOR('',#30089,1000.);
#7794=VECTOR('',#30092,1000.);
#7795=VECTOR('',#30093,1000.);
#7796=VECTOR('',#30096,1000.);
#7797=VECTOR('',#30097,1000.);
#7798=VECTOR('',#30118,1000.);
#7799=VECTOR('',#30119,1000.);
#7800=VECTOR('',#30122,1000.);
#7801=VECTOR('',#30123,1000.);
#7802=VECTOR('',#30126,1000.);
#7803=VECTOR('',#30127,1000.);
#7804=VECTOR('',#30130,1000.);
#7805=VECTOR('',#30131,1000.);
#7806=VECTOR('',#30136,1000.);
#7807=VECTOR('',#30137,1000.);
#7808=VECTOR('',#30140,1000.);
#7809=VECTOR('',#30141,1000.);
#7810=VECTOR('',#30164,1000.);
#9543=CIRCLE('',#26231,5.49999999999995);
#9544=CIRCLE('',#26232,5.49999999999995);
#9545=CIRCLE('',#26234,3.5);
#9546=CIRCLE('',#26236,3.49999999999995);
#9547=CIRCLE('',#26238,3.5);
#9548=CIRCLE('',#26239,3.49999999999995);
#9549=CIRCLE('',#26240,3.5);
#9550=CIRCLE('',#26242,3.49999999999995);
#9551=CIRCLE('',#26245,5.49999999999995);
#9552=CIRCLE('',#26246,5.49999999999995);
#9553=CIRCLE('',#26248,3.5);
#9554=CIRCLE('',#26250,3.49999999999995);
#9555=CIRCLE('',#26252,3.5);
#9556=CIRCLE('',#26253,3.49999999999995);
#9557=CIRCLE('',#26254,3.5);
#9558=CIRCLE('',#26256,3.49999999999995);
#9559=CIRCLE('',#26259,5.49999999999995);
#9560=CIRCLE('',#26260,5.49999999999995);
#9561=CIRCLE('',#26262,3.5);
#9562=CIRCLE('',#26264,3.49999999999995);
#9563=CIRCLE('',#26266,3.5);
#9564=CIRCLE('',#26267,3.49999999999995);
#9565=CIRCLE('',#26268,3.5);
#9566=CIRCLE('',#26270,3.49999999999995);
#9567=CIRCLE('',#26273,5.49999999999995);
#9568=CIRCLE('',#26274,5.49999999999995);
#9569=CIRCLE('',#26276,3.5);
#9570=CIRCLE('',#26278,3.49999999999995);
#9571=CIRCLE('',#26280,3.5);
#9572=CIRCLE('',#26281,3.49999999999995);
#9573=CIRCLE('',#26282,3.5);
#9574=CIRCLE('',#26284,3.49999999999995);
#9575=CIRCLE('',#26287,5.49999999999995);
#9576=CIRCLE('',#26288,5.49999999999995);
#9577=CIRCLE('',#26290,3.5);
#9578=CIRCLE('',#26292,3.49999999999995);
#9579=CIRCLE('',#26294,3.5);
#9580=CIRCLE('',#26295,3.49999999999995);
#9581=CIRCLE('',#26296,3.5);
#9582=CIRCLE('',#26298,3.49999999999995);
#9583=CIRCLE('',#26301,5.49999999999995);
#9584=CIRCLE('',#26302,5.49999999999995);
#9585=CIRCLE('',#26304,3.5);
#9586=CIRCLE('',#26306,3.49999999999995);
#9587=CIRCLE('',#26308,3.5);
#9588=CIRCLE('',#26309,3.49999999999995);
#9589=CIRCLE('',#26310,3.5);
#9590=CIRCLE('',#26312,3.49999999999995);
#9591=CIRCLE('',#26315,5.50000000000001);
#9592=CIRCLE('',#26316,5.50000000000001);
#9593=CIRCLE('',#26318,3.5);
#9594=CIRCLE('',#26320,3.5);
#9595=CIRCLE('',#26322,3.5);
#9596=CIRCLE('',#26323,3.5);
#9597=CIRCLE('',#26324,3.5);
#9598=CIRCLE('',#26326,3.5);
#9599=CIRCLE('',#26329,5.50000000000001);
#9600=CIRCLE('',#26330,5.50000000000001);
#9601=CIRCLE('',#26332,3.5);
#9602=CIRCLE('',#26334,3.5);
#9603=CIRCLE('',#26336,3.5);
#9604=CIRCLE('',#26337,3.5);
#9605=CIRCLE('',#26338,3.5);
#9606=CIRCLE('',#26340,3.5);
#9607=CIRCLE('',#26343,5.50000000000001);
#9608=CIRCLE('',#26344,5.50000000000001);
#9609=CIRCLE('',#26346,3.5);
#9610=CIRCLE('',#26348,3.5);
#9611=CIRCLE('',#26350,3.5);
#9612=CIRCLE('',#26351,3.5);
#9613=CIRCLE('',#26352,3.5);
#9614=CIRCLE('',#26354,3.5);
#9615=CIRCLE('',#26357,5.50000000000001);
#9616=CIRCLE('',#26358,5.50000000000001);
#9617=CIRCLE('',#26360,3.5);
#9618=CIRCLE('',#26362,3.5);
#9619=CIRCLE('',#26364,3.5);
#9620=CIRCLE('',#26365,3.5);
#9621=CIRCLE('',#26366,3.5);
#9622=CIRCLE('',#26368,3.5);
#9623=CIRCLE('',#26371,5.50000000000001);
#9624=CIRCLE('',#26372,5.50000000000001);
#9625=CIRCLE('',#26374,3.5);
#9626=CIRCLE('',#26376,3.5);
#9627=CIRCLE('',#26378,3.5);
#9628=CIRCLE('',#26379,3.5);
#9629=CIRCLE('',#26380,3.5);
#9630=CIRCLE('',#26382,3.5);
#9631=CIRCLE('',#26385,5.50000000000001);
#9632=CIRCLE('',#26386,5.50000000000001);
#9633=CIRCLE('',#26388,3.5);
#9634=CIRCLE('',#26390,3.5);
#9635=CIRCLE('',#26392,3.5);
#9636=CIRCLE('',#26393,3.5);
#9637=CIRCLE('',#26394,3.5);
#9638=CIRCLE('',#26396,3.5);
#9639=CIRCLE('',#26399,5.50000000000001);
#9640=CIRCLE('',#26400,5.50000000000001);
#9641=CIRCLE('',#26402,3.5);
#9642=CIRCLE('',#26404,3.49999999999999);
#9643=CIRCLE('',#26406,3.5);
#9644=CIRCLE('',#26407,3.5);
#9645=CIRCLE('',#26408,3.5);
#9646=CIRCLE('',#26410,3.49999999999999);
#9647=CIRCLE('',#26413,5.5);
#9648=CIRCLE('',#26414,5.5);
#9649=CIRCLE('',#26416,3.5);
#9650=CIRCLE('',#26418,3.5);
#9651=CIRCLE('',#26420,3.5);
#9652=CIRCLE('',#26421,3.5);
#9653=CIRCLE('',#26422,3.5);
#9654=CIRCLE('',#26424,3.5);
#9655=CIRCLE('',#26427,5.5);
#9656=CIRCLE('',#26428,5.5);
#9657=CIRCLE('',#26430,3.5);
#9658=CIRCLE('',#26432,3.49999999999999);
#9659=CIRCLE('',#26434,3.5);
#9660=CIRCLE('',#26435,3.5);
#9661=CIRCLE('',#26436,3.5);
#9662=CIRCLE('',#26438,3.49999999999999);
#9663=CIRCLE('',#26488,1.);
#9664=CIRCLE('',#26489,0.5);
#9665=CIRCLE('',#26490,0.5);
#9666=CIRCLE('',#26491,0.5);
#9667=CIRCLE('',#26492,2.3);
#9668=CIRCLE('',#26493,0.5);
#9669=CIRCLE('',#26494,0.5);
#9670=CIRCLE('',#26495,0.5);
#9671=CIRCLE('',#26496,0.5);
#9672=CIRCLE('',#26497,2.3);
#9673=CIRCLE('',#26498,0.5);
#9674=CIRCLE('',#26499,0.5);
#9675=CIRCLE('',#26500,2.3);
#9676=CIRCLE('',#26501,0.5);
#9677=CIRCLE('',#26502,0.5);
#9678=CIRCLE('',#26503,0.5);
#9679=CIRCLE('',#26504,0.5);
#9680=CIRCLE('',#26505,2.3);
#9681=CIRCLE('',#26506,0.5);
#9682=CIRCLE('',#26507,0.5);
#9683=CIRCLE('',#26508,0.5);
#9684=CIRCLE('',#26509,1.);
#9685=CIRCLE('',#26511,1.);
#9686=CIRCLE('',#26512,0.5);
#9687=CIRCLE('',#26513,0.5);
#9688=CIRCLE('',#26514,0.5);
#9689=CIRCLE('',#26515,2.3);
#9690=CIRCLE('',#26516,0.5);
#9691=CIRCLE('',#26517,0.5);
#9692=CIRCLE('',#26518,0.5);
#9693=CIRCLE('',#26519,0.5);
#9694=CIRCLE('',#26520,2.3);
#9695=CIRCLE('',#26521,0.5);
#9696=CIRCLE('',#26522,0.5);
#9697=CIRCLE('',#26523,2.3);
#9698=CIRCLE('',#26524,0.5);
#9699=CIRCLE('',#26525,0.5);
#9700=CIRCLE('',#26526,0.5);
#9701=CIRCLE('',#26527,0.5);
#9702=CIRCLE('',#26528,2.3);
#9703=CIRCLE('',#26529,0.5);
#9704=CIRCLE('',#26530,0.5);
#9705=CIRCLE('',#26531,0.5);
#9706=CIRCLE('',#26532,1.);
#10796=VERTEX_POINT('',#36678);
#10797=VERTEX_POINT('',#36680);
#10798=VERTEX_POINT('',#36684);
#10799=VERTEX_POINT('',#36685);
#10800=VERTEX_POINT('',#36687);
#10801=VERTEX_POINT('',#36689);
#10802=VERTEX_POINT('',#36691);
#10803=VERTEX_POINT('',#36693);
#10804=VERTEX_POINT('',#36695);
#10805=VERTEX_POINT('',#36698);
#10806=VERTEX_POINT('',#36700);
#10807=VERTEX_POINT('',#36702);
#10808=VERTEX_POINT('',#36706);
#10809=VERTEX_POINT('',#36708);
#10810=VERTEX_POINT('',#36712);
#10811=VERTEX_POINT('',#36713);
#10812=VERTEX_POINT('',#36715);
#10813=VERTEX_POINT('',#36717);
#10814=VERTEX_POINT('',#36719);
#10815=VERTEX_POINT('',#36721);
#10816=VERTEX_POINT('',#36723);
#10817=VERTEX_POINT('',#36726);
#10818=VERTEX_POINT('',#36728);
#10819=VERTEX_POINT('',#36730);
#10820=VERTEX_POINT('',#36734);
#10821=VERTEX_POINT('',#36736);
#10822=VERTEX_POINT('',#36740);
#10823=VERTEX_POINT('',#36741);
#10824=VERTEX_POINT('',#36743);
#10825=VERTEX_POINT('',#36745);
#10826=VERTEX_POINT('',#36747);
#10827=VERTEX_POINT('',#36749);
#10828=VERTEX_POINT('',#36751);
#10829=VERTEX_POINT('',#36754);
#10830=VERTEX_POINT('',#36756);
#10831=VERTEX_POINT('',#36758);
#10832=VERTEX_POINT('',#36762);
#10833=VERTEX_POINT('',#36764);
#10834=VERTEX_POINT('',#36768);
#10835=VERTEX_POINT('',#36769);
#10836=VERTEX_POINT('',#36771);
#10837=VERTEX_POINT('',#36773);
#10838=VERTEX_POINT('',#36775);
#10839=VERTEX_POINT('',#36777);
#10840=VERTEX_POINT('',#36779);
#10841=VERTEX_POINT('',#36782);
#10842=VERTEX_POINT('',#36784);
#10843=VERTEX_POINT('',#36786);
#10844=VERTEX_POINT('',#36790);
#10845=VERTEX_POINT('',#36792);
#10846=VERTEX_POINT('',#36796);
#10847=VERTEX_POINT('',#36797);
#10848=VERTEX_POINT('',#36799);
#10849=VERTEX_POINT('',#36801);
#10850=VERTEX_POINT('',#36803);
#10851=VERTEX_POINT('',#36805);
#10852=VERTEX_POINT('',#36807);
#10853=VERTEX_POINT('',#36810);
#10854=VERTEX_POINT('',#36812);
#10855=VERTEX_POINT('',#36814);
#10856=VERTEX_POINT('',#36818);
#10857=VERTEX_POINT('',#36820);
#10858=VERTEX_POINT('',#36824);
#10859=VERTEX_POINT('',#36825);
#10860=VERTEX_POINT('',#36827);
#10861=VERTEX_POINT('',#36829);
#10862=VERTEX_POINT('',#36831);
#10863=VERTEX_POINT('',#36833);
#10864=VERTEX_POINT('',#36835);
#10865=VERTEX_POINT('',#36838);
#10866=VERTEX_POINT('',#36840);
#10867=VERTEX_POINT('',#36842);
#10868=VERTEX_POINT('',#36846);
#10869=VERTEX_POINT('',#36848);
#10870=VERTEX_POINT('',#36852);
#10871=VERTEX_POINT('',#36853);
#10872=VERTEX_POINT('',#36855);
#10873=VERTEX_POINT('',#36857);
#10874=VERTEX_POINT('',#36859);
#10875=VERTEX_POINT('',#36861);
#10876=VERTEX_POINT('',#36863);
#10877=VERTEX_POINT('',#36866);
#10878=VERTEX_POINT('',#36868);
#10879=VERTEX_POINT('',#36870);
#10880=VERTEX_POINT('',#36874);
#10881=VERTEX_POINT('',#36876);
#10882=VERTEX_POINT('',#36880);
#10883=VERTEX_POINT('',#36881);
#10884=VERTEX_POINT('',#36883);
#10885=VERTEX_POINT('',#36885);
#10886=VERTEX_POINT('',#36887);
#10887=VERTEX_POINT('',#36889);
#10888=VERTEX_POINT('',#36891);
#10889=VERTEX_POINT('',#36894);
#10890=VERTEX_POINT('',#36896);
#10891=VERTEX_POINT('',#36898);
#10892=VERTEX_POINT('',#36902);
#10893=VERTEX_POINT('',#36904);
#10894=VERTEX_POINT('',#36908);
#10895=VERTEX_POINT('',#36909);
#10896=VERTEX_POINT('',#36911);
#10897=VERTEX_POINT('',#36913);
#10898=VERTEX_POINT('',#36915);
#10899=VERTEX_POINT('',#36917);
#10900=VERTEX_POINT('',#36919);
#10901=VERTEX_POINT('',#36922);
#10902=VERTEX_POINT('',#36924);
#10903=VERTEX_POINT('',#36926);
#10904=VERTEX_POINT('',#36930);
#10905=VERTEX_POINT('',#36932);
#10906=VERTEX_POINT('',#36936);
#10907=VERTEX_POINT('',#36937);
#10908=VERTEX_POINT('',#36939);
#10909=VERTEX_POINT('',#36941);
#10910=VERTEX_POINT('',#36943);
#10911=VERTEX_POINT('',#36945);
#10912=VERTEX_POINT('',#36947);
#10913=VERTEX_POINT('',#36950);
#10914=VERTEX_POINT('',#36952);
#10915=VERTEX_POINT('',#36954);
#10916=VERTEX_POINT('',#36958);
#10917=VERTEX_POINT('',#36960);
#10918=VERTEX_POINT('',#36964);
#10919=VERTEX_POINT('',#36965);
#10920=VERTEX_POINT('',#36967);
#10921=VERTEX_POINT('',#36969);
#10922=VERTEX_POINT('',#36971);
#10923=VERTEX_POINT('',#36973);
#10924=VERTEX_POINT('',#36975);
#10925=VERTEX_POINT('',#36978);
#10926=VERTEX_POINT('',#36980);
#10927=VERTEX_POINT('',#36982);
#10928=VERTEX_POINT('',#36986);
#10929=VERTEX_POINT('',#36988);
#10930=VERTEX_POINT('',#36992);
#10931=VERTEX_POINT('',#36993);
#10932=VERTEX_POINT('',#36995);
#10933=VERTEX_POINT('',#36997);
#10934=VERTEX_POINT('',#36999);
#10935=VERTEX_POINT('',#37001);
#10936=VERTEX_POINT('',#37003);
#10937=VERTEX_POINT('',#37006);
#10938=VERTEX_POINT('',#37008);
#10939=VERTEX_POINT('',#37010);
#10940=VERTEX_POINT('',#37014);
#10941=VERTEX_POINT('',#37016);
#10942=VERTEX_POINT('',#37020);
#10943=VERTEX_POINT('',#37021);
#10944=VERTEX_POINT('',#37023);
#10945=VERTEX_POINT('',#37025);
#10946=VERTEX_POINT('',#37027);
#10947=VERTEX_POINT('',#37029);
#10948=VERTEX_POINT('',#37031);
#10949=VERTEX_POINT('',#37034);
#10950=VERTEX_POINT('',#37036);
#10951=VERTEX_POINT('',#37038);
#10952=VERTEX_POINT('',#37042);
#10953=VERTEX_POINT('',#37044);
#10954=VERTEX_POINT('',#37048);
#10955=VERTEX_POINT('',#37049);
#10956=VERTEX_POINT('',#37051);
#10957=VERTEX_POINT('',#37053);
#10958=VERTEX_POINT('',#37055);
#10959=VERTEX_POINT('',#37057);
#10960=VERTEX_POINT('',#37059);
#10961=VERTEX_POINT('',#37062);
#10962=VERTEX_POINT('',#37064);
#10963=VERTEX_POINT('',#37066);
#10964=VERTEX_POINT('',#37070);
#10965=VERTEX_POINT('',#37072);
#10966=VERTEX_POINT('',#37076);
#10967=VERTEX_POINT('',#37077);
#10968=VERTEX_POINT('',#37079);
#10969=VERTEX_POINT('',#37081);
#10970=VERTEX_POINT('',#37083);
#10971=VERTEX_POINT('',#37085);
#10972=VERTEX_POINT('',#37087);
#10973=VERTEX_POINT('',#37090);
#10974=VERTEX_POINT('',#37092);
#10975=VERTEX_POINT('',#37094);
#10976=VERTEX_POINT('',#37098);
#10977=VERTEX_POINT('',#37100);
#10978=VERTEX_POINT('',#37121);
#10979=VERTEX_POINT('',#37123);
#10980=VERTEX_POINT('',#37125);
#10981=VERTEX_POINT('',#37131);
#10982=VERTEX_POINT('',#37133);
#10983=VERTEX_POINT('',#37135);
#10984=VERTEX_POINT('',#37137);
#10985=VERTEX_POINT('',#37219);
#10986=VERTEX_POINT('',#37221);
#10987=VERTEX_POINT('',#37228);
#10988=VERTEX_POINT('',#37230);
#10989=VERTEX_POINT('',#37232);
#10990=VERTEX_POINT('',#37234);
#10991=VERTEX_POINT('',#37236);
#10992=VERTEX_POINT('',#37238);
#10993=VERTEX_POINT('',#37240);
#10994=VERTEX_POINT('',#37242);
#10995=VERTEX_POINT('',#37244);
#10996=VERTEX_POINT('',#37246);
#10997=VERTEX_POINT('',#37248);
#10998=VERTEX_POINT('',#37250);
#10999=VERTEX_POINT('',#37252);
#11000=VERTEX_POINT('',#37254);
#11001=VERTEX_POINT('',#37256);
#11002=VERTEX_POINT('',#37258);
#11003=VERTEX_POINT('',#37260);
#11004=VERTEX_POINT('',#37262);
#11005=VERTEX_POINT('',#37264);
#11006=VERTEX_POINT('',#37266);
#11007=VERTEX_POINT('',#37268);
#11008=VERTEX_POINT('',#37270);
#11009=VERTEX_POINT('',#37272);
#11010=VERTEX_POINT('',#37274);
#11011=VERTEX_POINT('',#37276);
#11012=VERTEX_POINT('',#37278);
#11013=VERTEX_POINT('',#37280);
#11014=VERTEX_POINT('',#37282);
#11015=VERTEX_POINT('',#37284);
#11016=VERTEX_POINT('',#37286);
#11017=VERTEX_POINT('',#37288);
#11018=VERTEX_POINT('',#37290);
#11019=VERTEX_POINT('',#37292);
#11020=VERTEX_POINT('',#37294);
#11021=VERTEX_POINT('',#37296);
#11022=VERTEX_POINT('',#37298);
#11023=VERTEX_POINT('',#37300);
#11024=VERTEX_POINT('',#37302);
#11025=VERTEX_POINT('',#37304);
#11026=VERTEX_POINT('',#37306);
#11027=VERTEX_POINT('',#37309);
#11028=VERTEX_POINT('',#37314);
#11029=VERTEX_POINT('',#37316);
#11030=VERTEX_POINT('',#37318);
#11031=VERTEX_POINT('',#37320);
#11032=VERTEX_POINT('',#37322);
#11033=VERTEX_POINT('',#37324);
#11034=VERTEX_POINT('',#37326);
#11035=VERTEX_POINT('',#37328);
#11036=VERTEX_POINT('',#37330);
#11037=VERTEX_POINT('',#37332);
#11038=VERTEX_POINT('',#37334);
#11039=VERTEX_POINT('',#37336);
#11040=VERTEX_POINT('',#37338);
#11041=VERTEX_POINT('',#37340);
#11042=VERTEX_POINT('',#37342);
#11043=VERTEX_POINT('',#37344);
#11044=VERTEX_POINT('',#37346);
#11045=VERTEX_POINT('',#37348);
#11046=VERTEX_POINT('',#37350);
#11047=VERTEX_POINT('',#37352);
#11048=VERTEX_POINT('',#37354);
#11049=VERTEX_POINT('',#37356);
#11050=VERTEX_POINT('',#37358);
#11051=VERTEX_POINT('',#37360);
#11052=VERTEX_POINT('',#37362);
#11053=VERTEX_POINT('',#37364);
#11054=VERTEX_POINT('',#37366);
#11055=VERTEX_POINT('',#37368);
#11056=VERTEX_POINT('',#37370);
#11057=VERTEX_POINT('',#37372);
#11058=VERTEX_POINT('',#37374);
#11059=VERTEX_POINT('',#37376);
#11060=VERTEX_POINT('',#37378);
#11061=VERTEX_POINT('',#37380);
#11062=VERTEX_POINT('',#37382);
#11063=VERTEX_POINT('',#37384);
#11064=VERTEX_POINT('',#37386);
#11065=VERTEX_POINT('',#37388);
#11066=VERTEX_POINT('',#37390);
#11067=VERTEX_POINT('',#37392);
#13227=EDGE_CURVE('',#10796,#10796,#9543,.T.);
#13228=EDGE_CURVE('',#10796,#10797,#5638,.T.);
#13229=EDGE_CURVE('',#10797,#10797,#9544,.T.);
#13230=EDGE_CURVE('',#10798,#10799,#9545,.T.);
#13231=EDGE_CURVE('',#10800,#10798,#582,.T.);
#13232=EDGE_CURVE('',#10801,#10800,#9546,.T.);
#13233=EDGE_CURVE('',#10802,#10801,#583,.T.);
#13234=EDGE_CURVE('',#10803,#10802,#9547,.T.);
#13235=EDGE_CURVE('',#10803,#10804,#5639,.T.);
#13236=EDGE_CURVE('',#10804,#10804,#9548,.T.);
#13237=EDGE_CURVE('',#10805,#10803,#9549,.T.);
#13238=EDGE_CURVE('',#10806,#10805,#584,.T.);
#13239=EDGE_CURVE('',#10807,#10806,#9550,.T.);
#13240=EDGE_CURVE('',#10799,#10807,#585,.T.);
#13241=EDGE_CURVE('',#10808,#10808,#9551,.T.);
#13242=EDGE_CURVE('',#10808,#10809,#5640,.T.);
#13243=EDGE_CURVE('',#10809,#10809,#9552,.T.);
#13244=EDGE_CURVE('',#10810,#10811,#9553,.T.);
#13245=EDGE_CURVE('',#10812,#10810,#586,.T.);
#13246=EDGE_CURVE('',#10813,#10812,#9554,.T.);
#13247=EDGE_CURVE('',#10814,#10813,#587,.T.);
#13248=EDGE_CURVE('',#10815,#10814,#9555,.T.);
#13249=EDGE_CURVE('',#10815,#10816,#5641,.T.);
#13250=EDGE_CURVE('',#10816,#10816,#9556,.T.);
#13251=EDGE_CURVE('',#10817,#10815,#9557,.T.);
#13252=EDGE_CURVE('',#10818,#10817,#588,.T.);
#13253=EDGE_CURVE('',#10819,#10818,#9558,.T.);
#13254=EDGE_CURVE('',#10811,#10819,#589,.T.);
#13255=EDGE_CURVE('',#10820,#10820,#9559,.T.);
#13256=EDGE_CURVE('',#10820,#10821,#5642,.T.);
#13257=EDGE_CURVE('',#10821,#10821,#9560,.T.);
#13258=EDGE_CURVE('',#10822,#10823,#9561,.T.);
#13259=EDGE_CURVE('',#10824,#10822,#590,.T.);
#13260=EDGE_CURVE('',#10825,#10824,#9562,.T.);
#13261=EDGE_CURVE('',#10826,#10825,#591,.T.);
#13262=EDGE_CURVE('',#10827,#10826,#9563,.T.);
#13263=EDGE_CURVE('',#10827,#10828,#5643,.T.);
#13264=EDGE_CURVE('',#10828,#10828,#9564,.T.);
#13265=EDGE_CURVE('',#10829,#10827,#9565,.T.);
#13266=EDGE_CURVE('',#10830,#10829,#592,.T.);
#13267=EDGE_CURVE('',#10831,#10830,#9566,.T.);
#13268=EDGE_CURVE('',#10823,#10831,#593,.T.);
#13269=EDGE_CURVE('',#10832,#10832,#9567,.T.);
#13270=EDGE_CURVE('',#10832,#10833,#5644,.T.);
#13271=EDGE_CURVE('',#10833,#10833,#9568,.T.);
#13272=EDGE_CURVE('',#10834,#10835,#9569,.T.);
#13273=EDGE_CURVE('',#10836,#10834,#594,.T.);
#13274=EDGE_CURVE('',#10837,#10836,#9570,.T.);
#13275=EDGE_CURVE('',#10838,#10837,#595,.T.);
#13276=EDGE_CURVE('',#10839,#10838,#9571,.T.);
#13277=EDGE_CURVE('',#10839,#10840,#5645,.T.);
#13278=EDGE_CURVE('',#10840,#10840,#9572,.T.);
#13279=EDGE_CURVE('',#10841,#10839,#9573,.T.);
#13280=EDGE_CURVE('',#10842,#10841,#596,.T.);
#13281=EDGE_CURVE('',#10843,#10842,#9574,.T.);
#13282=EDGE_CURVE('',#10835,#10843,#597,.T.);
#13283=EDGE_CURVE('',#10844,#10844,#9575,.T.);
#13284=EDGE_CURVE('',#10844,#10845,#5646,.T.);
#13285=EDGE_CURVE('',#10845,#10845,#9576,.T.);
#13286=EDGE_CURVE('',#10846,#10847,#9577,.T.);
#13287=EDGE_CURVE('',#10848,#10846,#598,.T.);
#13288=EDGE_CURVE('',#10849,#10848,#9578,.T.);
#13289=EDGE_CURVE('',#10850,#10849,#599,.T.);
#13290=EDGE_CURVE('',#10851,#10850,#9579,.T.);
#13291=EDGE_CURVE('',#10851,#10852,#5647,.T.);
#13292=EDGE_CURVE('',#10852,#10852,#9580,.T.);
#13293=EDGE_CURVE('',#10853,#10851,#9581,.T.);
#13294=EDGE_CURVE('',#10854,#10853,#600,.T.);
#13295=EDGE_CURVE('',#10855,#10854,#9582,.T.);
#13296=EDGE_CURVE('',#10847,#10855,#601,.T.);
#13297=EDGE_CURVE('',#10856,#10856,#9583,.T.);
#13298=EDGE_CURVE('',#10856,#10857,#5648,.T.);
#13299=EDGE_CURVE('',#10857,#10857,#9584,.T.);
#13300=EDGE_CURVE('',#10858,#10859,#9585,.T.);
#13301=EDGE_CURVE('',#10860,#10858,#602,.T.);
#13302=EDGE_CURVE('',#10861,#10860,#9586,.T.);
#13303=EDGE_CURVE('',#10862,#10861,#603,.T.);
#13304=EDGE_CURVE('',#10863,#10862,#9587,.T.);
#13305=EDGE_CURVE('',#10863,#10864,#5649,.T.);
#13306=EDGE_CURVE('',#10864,#10864,#9588,.T.);
#13307=EDGE_CURVE('',#10865,#10863,#9589,.T.);
#13308=EDGE_CURVE('',#10866,#10865,#604,.T.);
#13309=EDGE_CURVE('',#10867,#10866,#9590,.T.);
#13310=EDGE_CURVE('',#10859,#10867,#605,.T.);
#13311=EDGE_CURVE('',#10868,#10868,#9591,.T.);
#13312=EDGE_CURVE('',#10868,#10869,#5650,.T.);
#13313=EDGE_CURVE('',#10869,#10869,#9592,.T.);
#13314=EDGE_CURVE('',#10870,#10871,#9593,.T.);
#13315=EDGE_CURVE('',#10872,#10870,#606,.T.);
#13316=EDGE_CURVE('',#10873,#10872,#9594,.T.);
#13317=EDGE_CURVE('',#10874,#10873,#607,.T.);
#13318=EDGE_CURVE('',#10875,#10874,#9595,.T.);
#13319=EDGE_CURVE('',#10875,#10876,#5651,.T.);
#13320=EDGE_CURVE('',#10876,#10876,#9596,.T.);
#13321=EDGE_CURVE('',#10877,#10875,#9597,.T.);
#13322=EDGE_CURVE('',#10878,#10877,#608,.T.);
#13323=EDGE_CURVE('',#10879,#10878,#9598,.T.);
#13324=EDGE_CURVE('',#10871,#10879,#609,.T.);
#13325=EDGE_CURVE('',#10880,#10880,#9599,.T.);
#13326=EDGE_CURVE('',#10880,#10881,#5652,.T.);
#13327=EDGE_CURVE('',#10881,#10881,#9600,.T.);
#13328=EDGE_CURVE('',#10882,#10883,#9601,.T.);
#13329=EDGE_CURVE('',#10884,#10882,#610,.T.);
#13330=EDGE_CURVE('',#10885,#10884,#9602,.T.);
#13331=EDGE_CURVE('',#10886,#10885,#611,.T.);
#13332=EDGE_CURVE('',#10887,#10886,#9603,.T.);
#13333=EDGE_CURVE('',#10887,#10888,#5653,.T.);
#13334=EDGE_CURVE('',#10888,#10888,#9604,.T.);
#13335=EDGE_CURVE('',#10889,#10887,#9605,.T.);
#13336=EDGE_CURVE('',#10890,#10889,#612,.T.);
#13337=EDGE_CURVE('',#10891,#10890,#9606,.T.);
#13338=EDGE_CURVE('',#10883,#10891,#613,.T.);
#13339=EDGE_CURVE('',#10892,#10892,#9607,.T.);
#13340=EDGE_CURVE('',#10892,#10893,#5654,.T.);
#13341=EDGE_CURVE('',#10893,#10893,#9608,.T.);
#13342=EDGE_CURVE('',#10894,#10895,#9609,.T.);
#13343=EDGE_CURVE('',#10896,#10894,#614,.T.);
#13344=EDGE_CURVE('',#10897,#10896,#9610,.T.);
#13345=EDGE_CURVE('',#10898,#10897,#615,.T.);
#13346=EDGE_CURVE('',#10899,#10898,#9611,.T.);
#13347=EDGE_CURVE('',#10899,#10900,#5655,.T.);
#13348=EDGE_CURVE('',#10900,#10900,#9612,.T.);
#13349=EDGE_CURVE('',#10901,#10899,#9613,.T.);
#13350=EDGE_CURVE('',#10902,#10901,#616,.T.);
#13351=EDGE_CURVE('',#10903,#10902,#9614,.T.);
#13352=EDGE_CURVE('',#10895,#10903,#617,.T.);
#13353=EDGE_CURVE('',#10904,#10904,#9615,.T.);
#13354=EDGE_CURVE('',#10904,#10905,#5656,.T.);
#13355=EDGE_CURVE('',#10905,#10905,#9616,.T.);
#13356=EDGE_CURVE('',#10906,#10907,#9617,.T.);
#13357=EDGE_CURVE('',#10908,#10906,#618,.T.);
#13358=EDGE_CURVE('',#10909,#10908,#9618,.T.);
#13359=EDGE_CURVE('',#10910,#10909,#619,.T.);
#13360=EDGE_CURVE('',#10911,#10910,#9619,.T.);
#13361=EDGE_CURVE('',#10911,#10912,#5657,.T.);
#13362=EDGE_CURVE('',#10912,#10912,#9620,.T.);
#13363=EDGE_CURVE('',#10913,#10911,#9621,.T.);
#13364=EDGE_CURVE('',#10914,#10913,#620,.T.);
#13365=EDGE_CURVE('',#10915,#10914,#9622,.T.);
#13366=EDGE_CURVE('',#10907,#10915,#621,.T.);
#13367=EDGE_CURVE('',#10916,#10916,#9623,.T.);
#13368=EDGE_CURVE('',#10916,#10917,#5658,.T.);
#13369=EDGE_CURVE('',#10917,#10917,#9624,.T.);
#13370=EDGE_CURVE('',#10918,#10919,#9625,.T.);
#13371=EDGE_CURVE('',#10920,#10918,#622,.T.);
#13372=EDGE_CURVE('',#10921,#10920,#9626,.T.);
#13373=EDGE_CURVE('',#10922,#10921,#623,.T.);
#13374=EDGE_CURVE('',#10923,#10922,#9627,.T.);
#13375=EDGE_CURVE('',#10923,#10924,#5659,.T.);
#13376=EDGE_CURVE('',#10924,#10924,#9628,.T.);
#13377=EDGE_CURVE('',#10925,#10923,#9629,.T.);
#13378=EDGE_CURVE('',#10926,#10925,#624,.T.);
#13379=EDGE_CURVE('',#10927,#10926,#9630,.T.);
#13380=EDGE_CURVE('',#10919,#10927,#625,.T.);
#13381=EDGE_CURVE('',#10928,#10928,#9631,.T.);
#13382=EDGE_CURVE('',#10928,#10929,#5660,.T.);
#13383=EDGE_CURVE('',#10929,#10929,#9632,.T.);
#13384=EDGE_CURVE('',#10930,#10931,#9633,.T.);
#13385=EDGE_CURVE('',#10932,#10930,#626,.T.);
#13386=EDGE_CURVE('',#10933,#10932,#9634,.T.);
#13387=EDGE_CURVE('',#10934,#10933,#627,.T.);
#13388=EDGE_CURVE('',#10935,#10934,#9635,.T.);
#13389=EDGE_CURVE('',#10935,#10936,#5661,.T.);
#13390=EDGE_CURVE('',#10936,#10936,#9636,.T.);
#13391=EDGE_CURVE('',#10937,#10935,#9637,.T.);
#13392=EDGE_CURVE('',#10938,#10937,#628,.T.);
#13393=EDGE_CURVE('',#10939,#10938,#9638,.T.);
#13394=EDGE_CURVE('',#10931,#10939,#629,.T.);
#13395=EDGE_CURVE('',#10940,#10940,#9639,.T.);
#13396=EDGE_CURVE('',#10940,#10941,#5662,.T.);
#13397=EDGE_CURVE('',#10941,#10941,#9640,.T.);
#13398=EDGE_CURVE('',#10942,#10943,#9641,.T.);
#13399=EDGE_CURVE('',#10944,#10942,#630,.T.);
#13400=EDGE_CURVE('',#10945,#10944,#9642,.T.);
#13401=EDGE_CURVE('',#10946,#10945,#631,.T.);
#13402=EDGE_CURVE('',#10947,#10946,#9643,.T.);
#13403=EDGE_CURVE('',#10947,#10948,#5663,.T.);
#13404=EDGE_CURVE('',#10948,#10948,#9644,.T.);
#13405=EDGE_CURVE('',#10949,#10947,#9645,.T.);
#13406=EDGE_CURVE('',#10950,#10949,#632,.T.);
#13407=EDGE_CURVE('',#10951,#10950,#9646,.T.);
#13408=EDGE_CURVE('',#10943,#10951,#633,.T.);
#13409=EDGE_CURVE('',#10952,#10952,#9647,.T.);
#13410=EDGE_CURVE('',#10952,#10953,#5664,.T.);
#13411=EDGE_CURVE('',#10953,#10953,#9648,.T.);
#13412=EDGE_CURVE('',#10954,#10955,#9649,.T.);
#13413=EDGE_CURVE('',#10956,#10954,#634,.T.);
#13414=EDGE_CURVE('',#10957,#10956,#9650,.T.);
#13415=EDGE_CURVE('',#10958,#10957,#635,.T.);
#13416=EDGE_CURVE('',#10959,#10958,#9651,.T.);
#13417=EDGE_CURVE('',#10959,#10960,#5665,.T.);
#13418=EDGE_CURVE('',#10960,#10960,#9652,.T.);
#13419=EDGE_CURVE('',#10961,#10959,#9653,.T.);
#13420=EDGE_CURVE('',#10962,#10961,#636,.T.);
#13421=EDGE_CURVE('',#10963,#10962,#9654,.T.);
#13422=EDGE_CURVE('',#10955,#10963,#637,.T.);
#13423=EDGE_CURVE('',#10964,#10964,#9655,.T.);
#13424=EDGE_CURVE('',#10964,#10965,#5666,.T.);
#13425=EDGE_CURVE('',#10965,#10965,#9656,.T.);
#13426=EDGE_CURVE('',#10966,#10967,#9657,.T.);
#13427=EDGE_CURVE('',#10968,#10966,#638,.T.);
#13428=EDGE_CURVE('',#10969,#10968,#9658,.T.);
#13429=EDGE_CURVE('',#10970,#10969,#639,.T.);
#13430=EDGE_CURVE('',#10971,#10970,#9659,.T.);
#13431=EDGE_CURVE('',#10971,#10972,#5667,.T.);
#13432=EDGE_CURVE('',#10972,#10972,#9660,.T.);
#13433=EDGE_CURVE('',#10973,#10971,#9661,.T.);
#13434=EDGE_CURVE('',#10974,#10973,#640,.T.);
#13435=EDGE_CURVE('',#10975,#10974,#9662,.T.);
#13436=EDGE_CURVE('',#10967,#10975,#641,.T.);
#13437=EDGE_CURVE('',#10976,#10802,#5668,.T.);
#13438=EDGE_CURVE('',#10977,#10801,#5669,.T.);
#13439=EDGE_CURVE('',#10976,#10977,#5670,.T.);
#13440=EDGE_CURVE('',#10799,#10817,#5671,.T.);
#13441=EDGE_CURVE('',#10807,#10818,#5672,.T.);
#13442=EDGE_CURVE('',#10800,#10813,#5673,.T.);
#13443=EDGE_CURVE('',#10812,#10825,#5674,.T.);
#13444=EDGE_CURVE('',#10824,#10837,#5675,.T.);
#13445=EDGE_CURVE('',#10836,#10849,#5676,.T.);
#13446=EDGE_CURVE('',#10848,#10861,#5677,.T.);
#13447=EDGE_CURVE('',#10860,#10873,#5678,.T.);
#13448=EDGE_CURVE('',#10872,#10885,#5679,.T.);
#13449=EDGE_CURVE('',#10884,#10897,#5680,.T.);
#13450=EDGE_CURVE('',#10896,#10909,#5681,.T.);
#13451=EDGE_CURVE('',#10908,#10921,#5682,.T.);
#13452=EDGE_CURVE('',#10920,#10933,#5683,.T.);
#13453=EDGE_CURVE('',#10932,#10945,#5684,.T.);
#13454=EDGE_CURVE('',#10944,#10957,#5685,.T.);
#13455=EDGE_CURVE('',#10956,#10969,#5686,.T.);
#13456=EDGE_CURVE('',#10968,#10978,#5687,.T.);
#13457=EDGE_CURVE('',#10979,#10978,#5688,.T.);
#13458=EDGE_CURVE('',#10980,#10979,#5689,.T.);
#13459=EDGE_CURVE('',#10980,#10977,#5690,.T.);
#13460=EDGE_CURVE('',#10798,#10814,#5691,.T.);
#13461=EDGE_CURVE('',#10981,#10806,#5692,.T.);
#13462=EDGE_CURVE('',#10981,#10982,#5693,.T.);
#13463=EDGE_CURVE('',#10982,#10983,#5694,.T.);
#13464=EDGE_CURVE('',#10984,#10983,#5695,.T.);
#13465=EDGE_CURVE('',#10975,#10984,#5696,.T.);
#13466=EDGE_CURVE('',#10963,#10974,#5697,.T.);
#13467=EDGE_CURVE('',#10951,#10962,#5698,.T.);
#13468=EDGE_CURVE('',#10939,#10950,#5699,.T.);
#13469=EDGE_CURVE('',#10927,#10938,#5700,.T.);
#13470=EDGE_CURVE('',#10915,#10926,#5701,.T.);
#13471=EDGE_CURVE('',#10903,#10914,#5702,.T.);
#13472=EDGE_CURVE('',#10891,#10902,#5703,.T.);
#13473=EDGE_CURVE('',#10879,#10890,#5704,.T.);
#13474=EDGE_CURVE('',#10867,#10878,#5705,.T.);
#13475=EDGE_CURVE('',#10855,#10866,#5706,.T.);
#13476=EDGE_CURVE('',#10843,#10854,#5707,.T.);
#13477=EDGE_CURVE('',#10831,#10842,#5708,.T.);
#13478=EDGE_CURVE('',#10819,#10830,#5709,.T.);
#13479=EDGE_CURVE('',#10810,#10826,#5710,.T.);
#13480=EDGE_CURVE('',#10811,#10829,#5711,.T.);
#13481=EDGE_CURVE('',#10822,#10838,#5712,.T.);
#13482=EDGE_CURVE('',#10823,#10841,#5713,.T.);
#13483=EDGE_CURVE('',#10834,#10850,#5714,.T.);
#13484=EDGE_CURVE('',#10835,#10853,#5715,.T.);
#13485=EDGE_CURVE('',#10846,#10862,#5716,.T.);
#13486=EDGE_CURVE('',#10847,#10865,#5717,.T.);
#13487=EDGE_CURVE('',#10858,#10874,#5718,.T.);
#13488=EDGE_CURVE('',#10859,#10877,#5719,.T.);
#13489=EDGE_CURVE('',#10870,#10886,#5720,.T.);
#13490=EDGE_CURVE('',#10871,#10889,#5721,.T.);
#13491=EDGE_CURVE('',#10882,#10898,#5722,.T.);
#13492=EDGE_CURVE('',#10883,#10901,#5723,.T.);
#13493=EDGE_CURVE('',#10894,#10910,#5724,.T.);
#13494=EDGE_CURVE('',#10895,#10913,#5725,.T.);
#13495=EDGE_CURVE('',#10906,#10922,#5726,.T.);
#13496=EDGE_CURVE('',#10907,#10925,#5727,.T.);
#13497=EDGE_CURVE('',#10918,#10934,#5728,.T.);
#13498=EDGE_CURVE('',#10919,#10937,#5729,.T.);
#13499=EDGE_CURVE('',#10930,#10946,#5730,.T.);
#13500=EDGE_CURVE('',#10931,#10949,#5731,.T.);
#13501=EDGE_CURVE('',#10942,#10958,#5732,.T.);
#13502=EDGE_CURVE('',#10943,#10961,#5733,.T.);
#13503=EDGE_CURVE('',#10954,#10970,#5734,.T.);
#13504=EDGE_CURVE('',#10955,#10973,#5735,.T.);
#13505=EDGE_CURVE('',#10966,#10985,#5736,.T.);
#13506=EDGE_CURVE('',#10967,#10986,#5737,.T.);
#13507=EDGE_CURVE('',#10986,#10985,#5738,.T.);
#13508=EDGE_CURVE('',#10984,#10986,#5739,.T.);
#13509=EDGE_CURVE('',#10987,#10980,#5740,.T.);
#13510=EDGE_CURVE('',#10988,#10987,#5741,.T.);
#13511=EDGE_CURVE('',#10988,#10989,#9663,.T.);
#13512=EDGE_CURVE('',#10990,#10989,#5742,.T.);
#13513=EDGE_CURVE('',#10990,#10991,#9664,.T.);
#13514=EDGE_CURVE('',#10992,#10991,#5743,.T.);
#13515=EDGE_CURVE('',#10992,#10993,#9665,.T.);
#13516=EDGE_CURVE('',#10994,#10993,#5744,.T.);
#13517=EDGE_CURVE('',#10994,#10995,#9666,.T.);
#13518=EDGE_CURVE('',#10995,#10996,#9667,.T.);
#13519=EDGE_CURVE('',#10996,#10997,#9668,.T.);
#13520=EDGE_CURVE('',#10998,#10997,#5745,.T.);
#13521=EDGE_CURVE('',#10998,#10999,#9669,.T.);
#13522=EDGE_CURVE('',#11000,#10999,#5746,.T.);
#13523=EDGE_CURVE('',#11000,#11001,#9670,.T.);
#13524=EDGE_CURVE('',#11002,#11001,#5747,.T.);
#13525=EDGE_CURVE('',#11002,#11003,#9671,.T.);
#13526=EDGE_CURVE('',#11003,#11004,#9672,.T.);
#13527=EDGE_CURVE('',#11004,#11005,#9673,.T.);
#13528=EDGE_CURVE('',#11006,#11005,#5748,.T.);
#13529=EDGE_CURVE('',#11007,#11006,#5749,.T.);
#13530=EDGE_CURVE('',#11007,#11008,#5750,.T.);
#13531=EDGE_CURVE('',#11008,#11009,#9674,.T.);
#13532=EDGE_CURVE('',#11010,#11009,#9675,.T.);
#13533=EDGE_CURVE('',#11010,#11011,#9676,.T.);
#13534=EDGE_CURVE('',#11011,#11012,#5751,.T.);
#13535=EDGE_CURVE('',#11012,#11013,#9677,.T.);
#13536=EDGE_CURVE('',#11013,#11014,#5752,.T.);
#13537=EDGE_CURVE('',#11014,#11015,#9678,.T.);
#13538=EDGE_CURVE('',#11015,#11016,#5753,.T.);
#13539=EDGE_CURVE('',#11016,#11017,#9679,.T.);
#13540=EDGE_CURVE('',#11018,#11017,#9680,.T.);
#13541=EDGE_CURVE('',#11018,#11019,#9681,.T.);
#13542=EDGE_CURVE('',#11019,#11020,#5754,.T.);
#13543=EDGE_CURVE('',#11020,#11021,#9682,.T.);
#13544=EDGE_CURVE('',#11021,#11022,#5755,.T.);
#13545=EDGE_CURVE('',#11022,#11023,#9683,.T.);
#13546=EDGE_CURVE('',#11023,#11024,#5756,.T.);
#13547=EDGE_CURVE('',#11024,#11025,#9684,.T.);
#13548=EDGE_CURVE('',#11025,#11026,#5757,.T.);
#13549=EDGE_CURVE('',#11026,#10982,#5758,.T.);
#13550=EDGE_CURVE('',#10981,#11027,#5759,.T.);
#13551=EDGE_CURVE('',#11027,#10976,#5760,.T.);
#13552=EDGE_CURVE('',#10985,#10978,#5761,.T.);
#13553=EDGE_CURVE('',#11028,#10983,#5762,.T.);
#13554=EDGE_CURVE('',#11029,#11028,#5763,.T.);
#13555=EDGE_CURVE('',#11029,#11030,#9685,.T.);
#13556=EDGE_CURVE('',#11031,#11030,#5764,.T.);
#13557=EDGE_CURVE('',#11031,#11032,#9686,.T.);
#13558=EDGE_CURVE('',#11033,#11032,#5765,.T.);
#13559=EDGE_CURVE('',#11033,#11034,#9687,.T.);
#13560=EDGE_CURVE('',#11035,#11034,#5766,.T.);
#13561=EDGE_CURVE('',#11035,#11036,#9688,.T.);
#13562=EDGE_CURVE('',#11036,#11037,#9689,.T.);
#13563=EDGE_CURVE('',#11037,#11038,#9690,.T.);
#13564=EDGE_CURVE('',#11039,#11038,#5767,.T.);
#13565=EDGE_CURVE('',#11039,#11040,#9691,.T.);
#13566=EDGE_CURVE('',#11041,#11040,#5768,.T.);
#13567=EDGE_CURVE('',#11041,#11042,#9692,.T.);
#13568=EDGE_CURVE('',#11043,#11042,#5769,.T.);
#13569=EDGE_CURVE('',#11043,#11044,#9693,.T.);
#13570=EDGE_CURVE('',#11044,#11045,#9694,.T.);
#13571=EDGE_CURVE('',#11045,#11046,#9695,.T.);
#13572=EDGE_CURVE('',#11047,#11046,#5770,.T.);
#13573=EDGE_CURVE('',#11047,#11048,#5771,.T.);
#13574=EDGE_CURVE('',#11048,#11049,#5772,.T.);
#13575=EDGE_CURVE('',#11049,#11050,#9696,.T.);
#13576=EDGE_CURVE('',#11051,#11050,#9697,.T.);
#13577=EDGE_CURVE('',#11051,#11052,#9698,.T.);
#13578=EDGE_CURVE('',#11052,#11053,#5773,.T.);
#13579=EDGE_CURVE('',#11053,#11054,#9699,.T.);
#13580=EDGE_CURVE('',#11054,#11055,#5774,.T.);
#13581=EDGE_CURVE('',#11055,#11056,#9700,.T.);
#13582=EDGE_CURVE('',#11056,#11057,#5775,.T.);
#13583=EDGE_CURVE('',#11057,#11058,#9701,.T.);
#13584=EDGE_CURVE('',#11059,#11058,#9702,.T.);
#13585=EDGE_CURVE('',#11059,#11060,#9703,.T.);
#13586=EDGE_CURVE('',#11060,#11061,#5776,.T.);
#13587=EDGE_CURVE('',#11061,#11062,#9704,.T.);
#13588=EDGE_CURVE('',#11062,#11063,#5777,.T.);
#13589=EDGE_CURVE('',#11063,#11064,#9705,.T.);
#13590=EDGE_CURVE('',#11064,#11065,#5778,.T.);
#13591=EDGE_CURVE('',#11065,#11066,#9706,.T.);
#13592=EDGE_CURVE('',#11066,#11067,#5779,.T.);
#13593=EDGE_CURVE('',#11067,#10979,#5780,.T.);
#13594=EDGE_CURVE('',#11034,#11020,#5781,.T.);
#13595=EDGE_CURVE('',#11019,#11035,#5782,.T.);
#13596=EDGE_CURVE('',#11015,#11039,#5783,.T.);
#13597=EDGE_CURVE('',#11038,#11016,#5784,.T.);
#13598=EDGE_CURVE('',#11011,#11043,#5785,.T.);
#13599=EDGE_CURVE('',#11042,#11012,#5786,.T.);
#13600=EDGE_CURVE('',#11046,#11008,#5787,.T.);
#13601=EDGE_CURVE('',#11007,#11047,#5788,.T.);
#13602=EDGE_CURVE('',#10993,#11061,#5789,.T.);
#13603=EDGE_CURVE('',#11060,#10994,#5790,.T.);
#13604=EDGE_CURVE('',#11052,#11002,#5791,.T.);
#13605=EDGE_CURVE('',#11001,#11053,#5792,.T.);
#13606=EDGE_CURVE('',#11006,#11048,#5793,.T.);
#13607=EDGE_CURVE('',#10987,#11067,#5794,.T.);
#13608=EDGE_CURVE('',#11066,#10988,#5795,.T.);
#13609=EDGE_CURVE('',#10989,#11065,#5796,.T.);
#13610=EDGE_CURVE('',#11064,#10990,#5797,.T.);
#13611=EDGE_CURVE('',#10991,#11063,#5798,.T.);
#13612=EDGE_CURVE('',#11062,#10992,#5799,.T.);
#13613=EDGE_CURVE('',#11056,#10998,#5800,.T.);
#13614=EDGE_CURVE('',#10997,#11057,#5801,.T.);
#13615=EDGE_CURVE('',#11054,#11000,#5802,.T.);
#13616=EDGE_CURVE('',#10999,#11055,#5803,.T.);
#13617=EDGE_CURVE('',#11005,#11049,#5804,.T.);
#13618=EDGE_CURVE('',#11003,#11051,#5805,.T.);
#13619=EDGE_CURVE('',#11050,#11004,#5806,.T.);
#13620=EDGE_CURVE('',#11058,#10996,#5807,.T.);
#13621=EDGE_CURVE('',#10995,#11059,#5808,.T.);
#13622=EDGE_CURVE('',#11013,#11041,#5809,.T.);
#13623=EDGE_CURVE('',#11040,#11014,#5810,.T.);
#13624=EDGE_CURVE('',#11032,#11022,#5811,.T.);
#13625=EDGE_CURVE('',#11021,#11033,#5812,.T.);
#13626=EDGE_CURVE('',#11030,#11024,#5813,.T.);
#13627=EDGE_CURVE('',#11023,#11031,#5814,.T.);
#13628=EDGE_CURVE('',#11025,#11029,#5815,.T.);
#13629=EDGE_CURVE('',#11026,#11028,#5816,.T.);
#13630=EDGE_CURVE('',#11044,#11010,#5817,.T.);
#13631=EDGE_CURVE('',#11009,#11045,#5818,.T.);
#13632=EDGE_CURVE('',#11017,#11037,#5819,.T.);
#13633=EDGE_CURVE('',#11036,#11018,#5820,.T.);
#13634=EDGE_CURVE('',#11027,#10805,#5821,.T.);
#17068=ORIENTED_EDGE('',*,*,#13227,.F.);
#17069=ORIENTED_EDGE('',*,*,#13228,.T.);
#17070=ORIENTED_EDGE('',*,*,#13229,.T.);
#17071=ORIENTED_EDGE('',*,*,#13228,.F.);
#17072=ORIENTED_EDGE('',*,*,#13230,.F.);
#17073=ORIENTED_EDGE('',*,*,#13231,.F.);
#17074=ORIENTED_EDGE('',*,*,#13232,.F.);
#17075=ORIENTED_EDGE('',*,*,#13233,.F.);
#17076=ORIENTED_EDGE('',*,*,#13234,.F.);
#17077=ORIENTED_EDGE('',*,*,#13235,.T.);
#17078=ORIENTED_EDGE('',*,*,#13236,.T.);
#17079=ORIENTED_EDGE('',*,*,#13235,.F.);
#17080=ORIENTED_EDGE('',*,*,#13237,.F.);
#17081=ORIENTED_EDGE('',*,*,#13238,.F.);
#17082=ORIENTED_EDGE('',*,*,#13239,.F.);
#17083=ORIENTED_EDGE('',*,*,#13240,.F.);
#17084=ORIENTED_EDGE('',*,*,#13241,.F.);
#17085=ORIENTED_EDGE('',*,*,#13242,.T.);
#17086=ORIENTED_EDGE('',*,*,#13243,.T.);
#17087=ORIENTED_EDGE('',*,*,#13242,.F.);
#17088=ORIENTED_EDGE('',*,*,#13244,.F.);
#17089=ORIENTED_EDGE('',*,*,#13245,.F.);
#17090=ORIENTED_EDGE('',*,*,#13246,.F.);
#17091=ORIENTED_EDGE('',*,*,#13247,.F.);
#17092=ORIENTED_EDGE('',*,*,#13248,.F.);
#17093=ORIENTED_EDGE('',*,*,#13249,.T.);
#17094=ORIENTED_EDGE('',*,*,#13250,.T.);
#17095=ORIENTED_EDGE('',*,*,#13249,.F.);
#17096=ORIENTED_EDGE('',*,*,#13251,.F.);
#17097=ORIENTED_EDGE('',*,*,#13252,.F.);
#17098=ORIENTED_EDGE('',*,*,#13253,.F.);
#17099=ORIENTED_EDGE('',*,*,#13254,.F.);
#17100=ORIENTED_EDGE('',*,*,#13255,.F.);
#17101=ORIENTED_EDGE('',*,*,#13256,.T.);
#17102=ORIENTED_EDGE('',*,*,#13257,.T.);
#17103=ORIENTED_EDGE('',*,*,#13256,.F.);
#17104=ORIENTED_EDGE('',*,*,#13258,.F.);
#17105=ORIENTED_EDGE('',*,*,#13259,.F.);
#17106=ORIENTED_EDGE('',*,*,#13260,.F.);
#17107=ORIENTED_EDGE('',*,*,#13261,.F.);
#17108=ORIENTED_EDGE('',*,*,#13262,.F.);
#17109=ORIENTED_EDGE('',*,*,#13263,.T.);
#17110=ORIENTED_EDGE('',*,*,#13264,.T.);
#17111=ORIENTED_EDGE('',*,*,#13263,.F.);
#17112=ORIENTED_EDGE('',*,*,#13265,.F.);
#17113=ORIENTED_EDGE('',*,*,#13266,.F.);
#17114=ORIENTED_EDGE('',*,*,#13267,.F.);
#17115=ORIENTED_EDGE('',*,*,#13268,.F.);
#17116=ORIENTED_EDGE('',*,*,#13269,.F.);
#17117=ORIENTED_EDGE('',*,*,#13270,.T.);
#17118=ORIENTED_EDGE('',*,*,#13271,.T.);
#17119=ORIENTED_EDGE('',*,*,#13270,.F.);
#17120=ORIENTED_EDGE('',*,*,#13272,.F.);
#17121=ORIENTED_EDGE('',*,*,#13273,.F.);
#17122=ORIENTED_EDGE('',*,*,#13274,.F.);
#17123=ORIENTED_EDGE('',*,*,#13275,.F.);
#17124=ORIENTED_EDGE('',*,*,#13276,.F.);
#17125=ORIENTED_EDGE('',*,*,#13277,.T.);
#17126=ORIENTED_EDGE('',*,*,#13278,.T.);
#17127=ORIENTED_EDGE('',*,*,#13277,.F.);
#17128=ORIENTED_EDGE('',*,*,#13279,.F.);
#17129=ORIENTED_EDGE('',*,*,#13280,.F.);
#17130=ORIENTED_EDGE('',*,*,#13281,.F.);
#17131=ORIENTED_EDGE('',*,*,#13282,.F.);
#17132=ORIENTED_EDGE('',*,*,#13283,.F.);
#17133=ORIENTED_EDGE('',*,*,#13284,.T.);
#17134=ORIENTED_EDGE('',*,*,#13285,.T.);
#17135=ORIENTED_EDGE('',*,*,#13284,.F.);
#17136=ORIENTED_EDGE('',*,*,#13286,.F.);
#17137=ORIENTED_EDGE('',*,*,#13287,.F.);
#17138=ORIENTED_EDGE('',*,*,#13288,.F.);
#17139=ORIENTED_EDGE('',*,*,#13289,.F.);
#17140=ORIENTED_EDGE('',*,*,#13290,.F.);
#17141=ORIENTED_EDGE('',*,*,#13291,.T.);
#17142=ORIENTED_EDGE('',*,*,#13292,.T.);
#17143=ORIENTED_EDGE('',*,*,#13291,.F.);
#17144=ORIENTED_EDGE('',*,*,#13293,.F.);
#17145=ORIENTED_EDGE('',*,*,#13294,.F.);
#17146=ORIENTED_EDGE('',*,*,#13295,.F.);
#17147=ORIENTED_EDGE('',*,*,#13296,.F.);
#17148=ORIENTED_EDGE('',*,*,#13297,.F.);
#17149=ORIENTED_EDGE('',*,*,#13298,.T.);
#17150=ORIENTED_EDGE('',*,*,#13299,.T.);
#17151=ORIENTED_EDGE('',*,*,#13298,.F.);
#17152=ORIENTED_EDGE('',*,*,#13300,.F.);
#17153=ORIENTED_EDGE('',*,*,#13301,.F.);
#17154=ORIENTED_EDGE('',*,*,#13302,.F.);
#17155=ORIENTED_EDGE('',*,*,#13303,.F.);
#17156=ORIENTED_EDGE('',*,*,#13304,.F.);
#17157=ORIENTED_EDGE('',*,*,#13305,.T.);
#17158=ORIENTED_EDGE('',*,*,#13306,.T.);
#17159=ORIENTED_EDGE('',*,*,#13305,.F.);
#17160=ORIENTED_EDGE('',*,*,#13307,.F.);
#17161=ORIENTED_EDGE('',*,*,#13308,.F.);
#17162=ORIENTED_EDGE('',*,*,#13309,.F.);
#17163=ORIENTED_EDGE('',*,*,#13310,.F.);
#17164=ORIENTED_EDGE('',*,*,#13311,.F.);
#17165=ORIENTED_EDGE('',*,*,#13312,.T.);
#17166=ORIENTED_EDGE('',*,*,#13313,.T.);
#17167=ORIENTED_EDGE('',*,*,#13312,.F.);
#17168=ORIENTED_EDGE('',*,*,#13314,.F.);
#17169=ORIENTED_EDGE('',*,*,#13315,.F.);
#17170=ORIENTED_EDGE('',*,*,#13316,.F.);
#17171=ORIENTED_EDGE('',*,*,#13317,.F.);
#17172=ORIENTED_EDGE('',*,*,#13318,.F.);
#17173=ORIENTED_EDGE('',*,*,#13319,.T.);
#17174=ORIENTED_EDGE('',*,*,#13320,.T.);
#17175=ORIENTED_EDGE('',*,*,#13319,.F.);
#17176=ORIENTED_EDGE('',*,*,#13321,.F.);
#17177=ORIENTED_EDGE('',*,*,#13322,.F.);
#17178=ORIENTED_EDGE('',*,*,#13323,.F.);
#17179=ORIENTED_EDGE('',*,*,#13324,.F.);
#17180=ORIENTED_EDGE('',*,*,#13325,.F.);
#17181=ORIENTED_EDGE('',*,*,#13326,.T.);
#17182=ORIENTED_EDGE('',*,*,#13327,.T.);
#17183=ORIENTED_EDGE('',*,*,#13326,.F.);
#17184=ORIENTED_EDGE('',*,*,#13328,.F.);
#17185=ORIENTED_EDGE('',*,*,#13329,.F.);
#17186=ORIENTED_EDGE('',*,*,#13330,.F.);
#17187=ORIENTED_EDGE('',*,*,#13331,.F.);
#17188=ORIENTED_EDGE('',*,*,#13332,.F.);
#17189=ORIENTED_EDGE('',*,*,#13333,.T.);
#17190=ORIENTED_EDGE('',*,*,#13334,.T.);
#17191=ORIENTED_EDGE('',*,*,#13333,.F.);
#17192=ORIENTED_EDGE('',*,*,#13335,.F.);
#17193=ORIENTED_EDGE('',*,*,#13336,.F.);
#17194=ORIENTED_EDGE('',*,*,#13337,.F.);
#17195=ORIENTED_EDGE('',*,*,#13338,.F.);
#17196=ORIENTED_EDGE('',*,*,#13339,.F.);
#17197=ORIENTED_EDGE('',*,*,#13340,.T.);
#17198=ORIENTED_EDGE('',*,*,#13341,.T.);
#17199=ORIENTED_EDGE('',*,*,#13340,.F.);
#17200=ORIENTED_EDGE('',*,*,#13342,.F.);
#17201=ORIENTED_EDGE('',*,*,#13343,.F.);
#17202=ORIENTED_EDGE('',*,*,#13344,.F.);
#17203=ORIENTED_EDGE('',*,*,#13345,.F.);
#17204=ORIENTED_EDGE('',*,*,#13346,.F.);
#17205=ORIENTED_EDGE('',*,*,#13347,.T.);
#17206=ORIENTED_EDGE('',*,*,#13348,.T.);
#17207=ORIENTED_EDGE('',*,*,#13347,.F.);
#17208=ORIENTED_EDGE('',*,*,#13349,.F.);
#17209=ORIENTED_EDGE('',*,*,#13350,.F.);
#17210=ORIENTED_EDGE('',*,*,#13351,.F.);
#17211=ORIENTED_EDGE('',*,*,#13352,.F.);
#17212=ORIENTED_EDGE('',*,*,#13353,.F.);
#17213=ORIENTED_EDGE('',*,*,#13354,.T.);
#17214=ORIENTED_EDGE('',*,*,#13355,.T.);
#17215=ORIENTED_EDGE('',*,*,#13354,.F.);
#17216=ORIENTED_EDGE('',*,*,#13356,.F.);
#17217=ORIENTED_EDGE('',*,*,#13357,.F.);
#17218=ORIENTED_EDGE('',*,*,#13358,.F.);
#17219=ORIENTED_EDGE('',*,*,#13359,.F.);
#17220=ORIENTED_EDGE('',*,*,#13360,.F.);
#17221=ORIENTED_EDGE('',*,*,#13361,.T.);
#17222=ORIENTED_EDGE('',*,*,#13362,.T.);
#17223=ORIENTED_EDGE('',*,*,#13361,.F.);
#17224=ORIENTED_EDGE('',*,*,#13363,.F.);
#17225=ORIENTED_EDGE('',*,*,#13364,.F.);
#17226=ORIENTED_EDGE('',*,*,#13365,.F.);
#17227=ORIENTED_EDGE('',*,*,#13366,.F.);
#17228=ORIENTED_EDGE('',*,*,#13367,.F.);
#17229=ORIENTED_EDGE('',*,*,#13368,.T.);
#17230=ORIENTED_EDGE('',*,*,#13369,.T.);
#17231=ORIENTED_EDGE('',*,*,#13368,.F.);
#17232=ORIENTED_EDGE('',*,*,#13370,.F.);
#17233=ORIENTED_EDGE('',*,*,#13371,.F.);
#17234=ORIENTED_EDGE('',*,*,#13372,.F.);
#17235=ORIENTED_EDGE('',*,*,#13373,.F.);
#17236=ORIENTED_EDGE('',*,*,#13374,.F.);
#17237=ORIENTED_EDGE('',*,*,#13375,.T.);
#17238=ORIENTED_EDGE('',*,*,#13376,.T.);
#17239=ORIENTED_EDGE('',*,*,#13375,.F.);
#17240=ORIENTED_EDGE('',*,*,#13377,.F.);
#17241=ORIENTED_EDGE('',*,*,#13378,.F.);
#17242=ORIENTED_EDGE('',*,*,#13379,.F.);
#17243=ORIENTED_EDGE('',*,*,#13380,.F.);
#17244=ORIENTED_EDGE('',*,*,#13381,.F.);
#17245=ORIENTED_EDGE('',*,*,#13382,.T.);
#17246=ORIENTED_EDGE('',*,*,#13383,.T.);
#17247=ORIENTED_EDGE('',*,*,#13382,.F.);
#17248=ORIENTED_EDGE('',*,*,#13384,.F.);
#17249=ORIENTED_EDGE('',*,*,#13385,.F.);
#17250=ORIENTED_EDGE('',*,*,#13386,.F.);
#17251=ORIENTED_EDGE('',*,*,#13387,.F.);
#17252=ORIENTED_EDGE('',*,*,#13388,.F.);
#17253=ORIENTED_EDGE('',*,*,#13389,.T.);
#17254=ORIENTED_EDGE('',*,*,#13390,.T.);
#17255=ORIENTED_EDGE('',*,*,#13389,.F.);
#17256=ORIENTED_EDGE('',*,*,#13391,.F.);
#17257=ORIENTED_EDGE('',*,*,#13392,.F.);
#17258=ORIENTED_EDGE('',*,*,#13393,.F.);
#17259=ORIENTED_EDGE('',*,*,#13394,.F.);
#17260=ORIENTED_EDGE('',*,*,#13395,.F.);
#17261=ORIENTED_EDGE('',*,*,#13396,.T.);
#17262=ORIENTED_EDGE('',*,*,#13397,.T.);
#17263=ORIENTED_EDGE('',*,*,#13396,.F.);
#17264=ORIENTED_EDGE('',*,*,#13398,.F.);
#17265=ORIENTED_EDGE('',*,*,#13399,.F.);
#17266=ORIENTED_EDGE('',*,*,#13400,.F.);
#17267=ORIENTED_EDGE('',*,*,#13401,.F.);
#17268=ORIENTED_EDGE('',*,*,#13402,.F.);
#17269=ORIENTED_EDGE('',*,*,#13403,.T.);
#17270=ORIENTED_EDGE('',*,*,#13404,.T.);
#17271=ORIENTED_EDGE('',*,*,#13403,.F.);
#17272=ORIENTED_EDGE('',*,*,#13405,.F.);
#17273=ORIENTED_EDGE('',*,*,#13406,.F.);
#17274=ORIENTED_EDGE('',*,*,#13407,.F.);
#17275=ORIENTED_EDGE('',*,*,#13408,.F.);
#17276=ORIENTED_EDGE('',*,*,#13409,.F.);
#17277=ORIENTED_EDGE('',*,*,#13410,.T.);
#17278=ORIENTED_EDGE('',*,*,#13411,.T.);
#17279=ORIENTED_EDGE('',*,*,#13410,.F.);
#17280=ORIENTED_EDGE('',*,*,#13412,.F.);
#17281=ORIENTED_EDGE('',*,*,#13413,.F.);
#17282=ORIENTED_EDGE('',*,*,#13414,.F.);
#17283=ORIENTED_EDGE('',*,*,#13415,.F.);
#17284=ORIENTED_EDGE('',*,*,#13416,.F.);
#17285=ORIENTED_EDGE('',*,*,#13417,.T.);
#17286=ORIENTED_EDGE('',*,*,#13418,.T.);
#17287=ORIENTED_EDGE('',*,*,#13417,.F.);
#17288=ORIENTED_EDGE('',*,*,#13419,.F.);
#17289=ORIENTED_EDGE('',*,*,#13420,.F.);
#17290=ORIENTED_EDGE('',*,*,#13421,.F.);
#17291=ORIENTED_EDGE('',*,*,#13422,.F.);
#17292=ORIENTED_EDGE('',*,*,#13423,.F.);
#17293=ORIENTED_EDGE('',*,*,#13424,.T.);
#17294=ORIENTED_EDGE('',*,*,#13425,.T.);
#17295=ORIENTED_EDGE('',*,*,#13424,.F.);
#17296=ORIENTED_EDGE('',*,*,#13426,.F.);
#17297=ORIENTED_EDGE('',*,*,#13427,.F.);
#17298=ORIENTED_EDGE('',*,*,#13428,.F.);
#17299=ORIENTED_EDGE('',*,*,#13429,.F.);
#17300=ORIENTED_EDGE('',*,*,#13430,.F.);
#17301=ORIENTED_EDGE('',*,*,#13431,.T.);
#17302=ORIENTED_EDGE('',*,*,#13432,.T.);
#17303=ORIENTED_EDGE('',*,*,#13431,.F.);
#17304=ORIENTED_EDGE('',*,*,#13433,.F.);
#17305=ORIENTED_EDGE('',*,*,#13434,.F.);
#17306=ORIENTED_EDGE('',*,*,#13435,.F.);
#17307=ORIENTED_EDGE('',*,*,#13436,.F.);
#17308=ORIENTED_EDGE('',*,*,#13437,.T.);
#17309=ORIENTED_EDGE('',*,*,#13233,.T.);
#17310=ORIENTED_EDGE('',*,*,#13438,.F.);
#17311=ORIENTED_EDGE('',*,*,#13439,.F.);
#17312=ORIENTED_EDGE('',*,*,#13440,.F.);
#17313=ORIENTED_EDGE('',*,*,#13240,.T.);
#17314=ORIENTED_EDGE('',*,*,#13441,.T.);
#17315=ORIENTED_EDGE('',*,*,#13252,.T.);
#17316=ORIENTED_EDGE('',*,*,#13438,.T.);
#17317=ORIENTED_EDGE('',*,*,#13232,.T.);
#17318=ORIENTED_EDGE('',*,*,#13442,.T.);
#17319=ORIENTED_EDGE('',*,*,#13246,.T.);
#17320=ORIENTED_EDGE('',*,*,#13443,.T.);
#17321=ORIENTED_EDGE('',*,*,#13260,.T.);
#17322=ORIENTED_EDGE('',*,*,#13444,.T.);
#17323=ORIENTED_EDGE('',*,*,#13274,.T.);
#17324=ORIENTED_EDGE('',*,*,#13445,.T.);
#17325=ORIENTED_EDGE('',*,*,#13288,.T.);
#17326=ORIENTED_EDGE('',*,*,#13446,.T.);
#17327=ORIENTED_EDGE('',*,*,#13302,.T.);
#17328=ORIENTED_EDGE('',*,*,#13447,.T.);
#17329=ORIENTED_EDGE('',*,*,#13316,.T.);
#17330=ORIENTED_EDGE('',*,*,#13448,.T.);
#17331=ORIENTED_EDGE('',*,*,#13330,.T.);
#17332=ORIENTED_EDGE('',*,*,#13449,.T.);
#17333=ORIENTED_EDGE('',*,*,#13344,.T.);
#17334=ORIENTED_EDGE('',*,*,#13450,.T.);
#17335=ORIENTED_EDGE('',*,*,#13358,.T.);
#17336=ORIENTED_EDGE('',*,*,#13451,.T.);
#17337=ORIENTED_EDGE('',*,*,#13372,.T.);
#17338=ORIENTED_EDGE('',*,*,#13452,.T.);
#17339=ORIENTED_EDGE('',*,*,#13386,.T.);
#17340=ORIENTED_EDGE('',*,*,#13453,.T.);
#17341=ORIENTED_EDGE('',*,*,#13400,.T.);
#17342=ORIENTED_EDGE('',*,*,#13454,.T.);
#17343=ORIENTED_EDGE('',*,*,#13414,.T.);
#17344=ORIENTED_EDGE('',*,*,#13455,.T.);
#17345=ORIENTED_EDGE('',*,*,#13428,.T.);
#17346=ORIENTED_EDGE('',*,*,#13456,.T.);
#17347=ORIENTED_EDGE('',*,*,#13457,.F.);
#17348=ORIENTED_EDGE('',*,*,#13458,.F.);
#17349=ORIENTED_EDGE('',*,*,#13459,.T.);
#17350=ORIENTED_EDGE('',*,*,#13460,.F.);
#17351=ORIENTED_EDGE('',*,*,#13230,.T.);
#17352=ORIENTED_EDGE('',*,*,#13440,.T.);
#17353=ORIENTED_EDGE('',*,*,#13251,.T.);
#17354=ORIENTED_EDGE('',*,*,#13248,.T.);
#17355=ORIENTED_EDGE('',*,*,#13441,.F.);
#17356=ORIENTED_EDGE('',*,*,#13239,.T.);
#17357=ORIENTED_EDGE('',*,*,#13461,.F.);
#17358=ORIENTED_EDGE('',*,*,#13462,.T.);
#17359=ORIENTED_EDGE('',*,*,#13463,.T.);
#17360=ORIENTED_EDGE('',*,*,#13464,.F.);
#17361=ORIENTED_EDGE('',*,*,#13465,.F.);
#17362=ORIENTED_EDGE('',*,*,#13435,.T.);
#17363=ORIENTED_EDGE('',*,*,#13466,.F.);
#17364=ORIENTED_EDGE('',*,*,#13421,.T.);
#17365=ORIENTED_EDGE('',*,*,#13467,.F.);
#17366=ORIENTED_EDGE('',*,*,#13407,.T.);
#17367=ORIENTED_EDGE('',*,*,#13468,.F.);
#17368=ORIENTED_EDGE('',*,*,#13393,.T.);
#17369=ORIENTED_EDGE('',*,*,#13469,.F.);
#17370=ORIENTED_EDGE('',*,*,#13379,.T.);
#17371=ORIENTED_EDGE('',*,*,#13470,.F.);
#17372=ORIENTED_EDGE('',*,*,#13365,.T.);
#17373=ORIENTED_EDGE('',*,*,#13471,.F.);
#17374=ORIENTED_EDGE('',*,*,#13351,.T.);
#17375=ORIENTED_EDGE('',*,*,#13472,.F.);
#17376=ORIENTED_EDGE('',*,*,#13337,.T.);
#17377=ORIENTED_EDGE('',*,*,#13473,.F.);
#17378=ORIENTED_EDGE('',*,*,#13323,.T.);
#17379=ORIENTED_EDGE('',*,*,#13474,.F.);
#17380=ORIENTED_EDGE('',*,*,#13309,.T.);
#17381=ORIENTED_EDGE('',*,*,#13475,.F.);
#17382=ORIENTED_EDGE('',*,*,#13295,.T.);
#17383=ORIENTED_EDGE('',*,*,#13476,.F.);
#17384=ORIENTED_EDGE('',*,*,#13281,.T.);
#17385=ORIENTED_EDGE('',*,*,#13477,.F.);
#17386=ORIENTED_EDGE('',*,*,#13267,.T.);
#17387=ORIENTED_EDGE('',*,*,#13478,.F.);
#17388=ORIENTED_EDGE('',*,*,#13253,.T.);
#17389=ORIENTED_EDGE('',*,*,#13442,.F.);
#17390=ORIENTED_EDGE('',*,*,#13231,.T.);
#17391=ORIENTED_EDGE('',*,*,#13460,.T.);
#17392=ORIENTED_EDGE('',*,*,#13247,.T.);
#17393=ORIENTED_EDGE('',*,*,#13479,.F.);
#17394=ORIENTED_EDGE('',*,*,#13244,.T.);
#17395=ORIENTED_EDGE('',*,*,#13480,.T.);
#17396=ORIENTED_EDGE('',*,*,#13265,.T.);
#17397=ORIENTED_EDGE('',*,*,#13262,.T.);
#17398=ORIENTED_EDGE('',*,*,#13480,.F.);
#17399=ORIENTED_EDGE('',*,*,#13254,.T.);
#17400=ORIENTED_EDGE('',*,*,#13478,.T.);
#17401=ORIENTED_EDGE('',*,*,#13266,.T.);
#17402=ORIENTED_EDGE('',*,*,#13443,.F.);
#17403=ORIENTED_EDGE('',*,*,#13245,.T.);
#17404=ORIENTED_EDGE('',*,*,#13479,.T.);
#17405=ORIENTED_EDGE('',*,*,#13261,.T.);
#17406=ORIENTED_EDGE('',*,*,#13481,.F.);
#17407=ORIENTED_EDGE('',*,*,#13258,.T.);
#17408=ORIENTED_EDGE('',*,*,#13482,.T.);
#17409=ORIENTED_EDGE('',*,*,#13279,.T.);
#17410=ORIENTED_EDGE('',*,*,#13276,.T.);
#17411=ORIENTED_EDGE('',*,*,#13482,.F.);
#17412=ORIENTED_EDGE('',*,*,#13268,.T.);
#17413=ORIENTED_EDGE('',*,*,#13477,.T.);
#17414=ORIENTED_EDGE('',*,*,#13280,.T.);
#17415=ORIENTED_EDGE('',*,*,#13444,.F.);
#17416=ORIENTED_EDGE('',*,*,#13259,.T.);
#17417=ORIENTED_EDGE('',*,*,#13481,.T.);
#17418=ORIENTED_EDGE('',*,*,#13275,.T.);
#17419=ORIENTED_EDGE('',*,*,#13483,.F.);
#17420=ORIENTED_EDGE('',*,*,#13272,.T.);
#17421=ORIENTED_EDGE('',*,*,#13484,.T.);
#17422=ORIENTED_EDGE('',*,*,#13293,.T.);
#17423=ORIENTED_EDGE('',*,*,#13290,.T.);
#17424=ORIENTED_EDGE('',*,*,#13484,.F.);
#17425=ORIENTED_EDGE('',*,*,#13282,.T.);
#17426=ORIENTED_EDGE('',*,*,#13476,.T.);
#17427=ORIENTED_EDGE('',*,*,#13294,.T.);
#17428=ORIENTED_EDGE('',*,*,#13445,.F.);
#17429=ORIENTED_EDGE('',*,*,#13273,.T.);
#17430=ORIENTED_EDGE('',*,*,#13483,.T.);
#17431=ORIENTED_EDGE('',*,*,#13289,.T.);
#17432=ORIENTED_EDGE('',*,*,#13485,.F.);
#17433=ORIENTED_EDGE('',*,*,#13286,.T.);
#17434=ORIENTED_EDGE('',*,*,#13486,.T.);
#17435=ORIENTED_EDGE('',*,*,#13307,.T.);
#17436=ORIENTED_EDGE('',*,*,#13304,.T.);
#17437=ORIENTED_EDGE('',*,*,#13486,.F.);
#17438=ORIENTED_EDGE('',*,*,#13296,.T.);
#17439=ORIENTED_EDGE('',*,*,#13475,.T.);
#17440=ORIENTED_EDGE('',*,*,#13308,.T.);
#17441=ORIENTED_EDGE('',*,*,#13446,.F.);
#17442=ORIENTED_EDGE('',*,*,#13287,.T.);
#17443=ORIENTED_EDGE('',*,*,#13485,.T.);
#17444=ORIENTED_EDGE('',*,*,#13303,.T.);
#17445=ORIENTED_EDGE('',*,*,#13487,.F.);
#17446=ORIENTED_EDGE('',*,*,#13300,.T.);
#17447=ORIENTED_EDGE('',*,*,#13488,.T.);
#17448=ORIENTED_EDGE('',*,*,#13321,.T.);
#17449=ORIENTED_EDGE('',*,*,#13318,.T.);
#17450=ORIENTED_EDGE('',*,*,#13488,.F.);
#17451=ORIENTED_EDGE('',*,*,#13310,.T.);
#17452=ORIENTED_EDGE('',*,*,#13474,.T.);
#17453=ORIENTED_EDGE('',*,*,#13322,.T.);
#17454=ORIENTED_EDGE('',*,*,#13447,.F.);
#17455=ORIENTED_EDGE('',*,*,#13301,.T.);
#17456=ORIENTED_EDGE('',*,*,#13487,.T.);
#17457=ORIENTED_EDGE('',*,*,#13317,.T.);
#17458=ORIENTED_EDGE('',*,*,#13489,.F.);
#17459=ORIENTED_EDGE('',*,*,#13314,.T.);
#17460=ORIENTED_EDGE('',*,*,#13490,.T.);
#17461=ORIENTED_EDGE('',*,*,#13335,.T.);
#17462=ORIENTED_EDGE('',*,*,#13332,.T.);
#17463=ORIENTED_EDGE('',*,*,#13490,.F.);
#17464=ORIENTED_EDGE('',*,*,#13324,.T.);
#17465=ORIENTED_EDGE('',*,*,#13473,.T.);
#17466=ORIENTED_EDGE('',*,*,#13336,.T.);
#17467=ORIENTED_EDGE('',*,*,#13448,.F.);
#17468=ORIENTED_EDGE('',*,*,#13315,.T.);
#17469=ORIENTED_EDGE('',*,*,#13489,.T.);
#17470=ORIENTED_EDGE('',*,*,#13331,.T.);
#17471=ORIENTED_EDGE('',*,*,#13491,.F.);
#17472=ORIENTED_EDGE('',*,*,#13328,.T.);
#17473=ORIENTED_EDGE('',*,*,#13492,.T.);
#17474=ORIENTED_EDGE('',*,*,#13349,.T.);
#17475=ORIENTED_EDGE('',*,*,#13346,.T.);
#17476=ORIENTED_EDGE('',*,*,#13492,.F.);
#17477=ORIENTED_EDGE('',*,*,#13338,.T.);
#17478=ORIENTED_EDGE('',*,*,#13472,.T.);
#17479=ORIENTED_EDGE('',*,*,#13350,.T.);
#17480=ORIENTED_EDGE('',*,*,#13449,.F.);
#17481=ORIENTED_EDGE('',*,*,#13329,.T.);
#17482=ORIENTED_EDGE('',*,*,#13491,.T.);
#17483=ORIENTED_EDGE('',*,*,#13345,.T.);
#17484=ORIENTED_EDGE('',*,*,#13493,.F.);
#17485=ORIENTED_EDGE('',*,*,#13342,.T.);
#17486=ORIENTED_EDGE('',*,*,#13494,.T.);
#17487=ORIENTED_EDGE('',*,*,#13363,.T.);
#17488=ORIENTED_EDGE('',*,*,#13360,.T.);
#17489=ORIENTED_EDGE('',*,*,#13494,.F.);
#17490=ORIENTED_EDGE('',*,*,#13352,.T.);
#17491=ORIENTED_EDGE('',*,*,#13471,.T.);
#17492=ORIENTED_EDGE('',*,*,#13364,.T.);
#17493=ORIENTED_EDGE('',*,*,#13450,.F.);
#17494=ORIENTED_EDGE('',*,*,#13343,.T.);
#17495=ORIENTED_EDGE('',*,*,#13493,.T.);
#17496=ORIENTED_EDGE('',*,*,#13359,.T.);
#17497=ORIENTED_EDGE('',*,*,#13495,.F.);
#17498=ORIENTED_EDGE('',*,*,#13356,.T.);
#17499=ORIENTED_EDGE('',*,*,#13496,.T.);
#17500=ORIENTED_EDGE('',*,*,#13377,.T.);
#17501=ORIENTED_EDGE('',*,*,#13374,.T.);
#17502=ORIENTED_EDGE('',*,*,#13496,.F.);
#17503=ORIENTED_EDGE('',*,*,#13366,.T.);
#17504=ORIENTED_EDGE('',*,*,#13470,.T.);
#17505=ORIENTED_EDGE('',*,*,#13378,.T.);
#17506=ORIENTED_EDGE('',*,*,#13497,.F.);
#17507=ORIENTED_EDGE('',*,*,#13370,.T.);
#17508=ORIENTED_EDGE('',*,*,#13498,.T.);
#17509=ORIENTED_EDGE('',*,*,#13391,.T.);
#17510=ORIENTED_EDGE('',*,*,#13388,.T.);
#17511=ORIENTED_EDGE('',*,*,#13451,.F.);
#17512=ORIENTED_EDGE('',*,*,#13357,.T.);
#17513=ORIENTED_EDGE('',*,*,#13495,.T.);
#17514=ORIENTED_EDGE('',*,*,#13373,.T.);
#17515=ORIENTED_EDGE('',*,*,#13498,.F.);
#17516=ORIENTED_EDGE('',*,*,#13380,.T.);
#17517=ORIENTED_EDGE('',*,*,#13469,.T.);
#17518=ORIENTED_EDGE('',*,*,#13392,.T.);
#17519=ORIENTED_EDGE('',*,*,#13452,.F.);
#17520=ORIENTED_EDGE('',*,*,#13371,.T.);
#17521=ORIENTED_EDGE('',*,*,#13497,.T.);
#17522=ORIENTED_EDGE('',*,*,#13387,.T.);
#17523=ORIENTED_EDGE('',*,*,#13499,.F.);
#17524=ORIENTED_EDGE('',*,*,#13384,.T.);
#17525=ORIENTED_EDGE('',*,*,#13500,.T.);
#17526=ORIENTED_EDGE('',*,*,#13405,.T.);
#17527=ORIENTED_EDGE('',*,*,#13402,.T.);
#17528=ORIENTED_EDGE('',*,*,#13500,.F.);
#17529=ORIENTED_EDGE('',*,*,#13394,.T.);
#17530=ORIENTED_EDGE('',*,*,#13468,.T.);
#17531=ORIENTED_EDGE('',*,*,#13406,.T.);
#17532=ORIENTED_EDGE('',*,*,#13453,.F.);
#17533=ORIENTED_EDGE('',*,*,#13385,.T.);
#17534=ORIENTED_EDGE('',*,*,#13499,.T.);
#17535=ORIENTED_EDGE('',*,*,#13401,.T.);
#17536=ORIENTED_EDGE('',*,*,#13501,.F.);
#17537=ORIENTED_EDGE('',*,*,#13398,.T.);
#17538=ORIENTED_EDGE('',*,*,#13502,.T.);
#17539=ORIENTED_EDGE('',*,*,#13419,.T.);
#17540=ORIENTED_EDGE('',*,*,#13416,.T.);
#17541=ORIENTED_EDGE('',*,*,#13502,.F.);
#17542=ORIENTED_EDGE('',*,*,#13408,.T.);
#17543=ORIENTED_EDGE('',*,*,#13467,.T.);
#17544=ORIENTED_EDGE('',*,*,#13420,.T.);
#17545=ORIENTED_EDGE('',*,*,#13503,.F.);
#17546=ORIENTED_EDGE('',*,*,#13412,.T.);
#17547=ORIENTED_EDGE('',*,*,#13504,.T.);
#17548=ORIENTED_EDGE('',*,*,#13433,.T.);
#17549=ORIENTED_EDGE('',*,*,#13430,.T.);
#17550=ORIENTED_EDGE('',*,*,#13454,.F.);
#17551=ORIENTED_EDGE('',*,*,#13399,.T.);
#17552=ORIENTED_EDGE('',*,*,#13501,.T.);
#17553=ORIENTED_EDGE('',*,*,#13415,.T.);
#17554=ORIENTED_EDGE('',*,*,#13504,.F.);
#17555=ORIENTED_EDGE('',*,*,#13422,.T.);
#17556=ORIENTED_EDGE('',*,*,#13466,.T.);
#17557=ORIENTED_EDGE('',*,*,#13434,.T.);
#17558=ORIENTED_EDGE('',*,*,#13505,.F.);
#17559=ORIENTED_EDGE('',*,*,#13426,.T.);
#17560=ORIENTED_EDGE('',*,*,#13506,.T.);
#17561=ORIENTED_EDGE('',*,*,#13507,.T.);
#17562=ORIENTED_EDGE('',*,*,#13455,.F.);
#17563=ORIENTED_EDGE('',*,*,#13413,.T.);
#17564=ORIENTED_EDGE('',*,*,#13503,.T.);
#17565=ORIENTED_EDGE('',*,*,#13429,.T.);
#17566=ORIENTED_EDGE('',*,*,#13506,.F.);
#17567=ORIENTED_EDGE('',*,*,#13436,.T.);
#17568=ORIENTED_EDGE('',*,*,#13465,.T.);
#17569=ORIENTED_EDGE('',*,*,#13508,.T.);
#17570=ORIENTED_EDGE('',*,*,#13439,.T.);
#17571=ORIENTED_EDGE('',*,*,#13459,.F.);
#17572=ORIENTED_EDGE('',*,*,#13509,.F.);
#17573=ORIENTED_EDGE('',*,*,#13510,.F.);
#17574=ORIENTED_EDGE('',*,*,#13511,.T.);
#17575=ORIENTED_EDGE('',*,*,#13512,.F.);
#17576=ORIENTED_EDGE('',*,*,#13513,.T.);
#17577=ORIENTED_EDGE('',*,*,#13514,.F.);
#17578=ORIENTED_EDGE('',*,*,#13515,.T.);
#17579=ORIENTED_EDGE('',*,*,#13516,.F.);
#17580=ORIENTED_EDGE('',*,*,#13517,.T.);
#17581=ORIENTED_EDGE('',*,*,#13518,.T.);
#17582=ORIENTED_EDGE('',*,*,#13519,.T.);
#17583=ORIENTED_EDGE('',*,*,#13520,.F.);
#17584=ORIENTED_EDGE('',*,*,#13521,.T.);
#17585=ORIENTED_EDGE('',*,*,#13522,.F.);
#17586=ORIENTED_EDGE('',*,*,#13523,.T.);
#17587=ORIENTED_EDGE('',*,*,#13524,.F.);
#17588=ORIENTED_EDGE('',*,*,#13525,.T.);
#17589=ORIENTED_EDGE('',*,*,#13526,.T.);
#17590=ORIENTED_EDGE('',*,*,#13527,.T.);
#17591=ORIENTED_EDGE('',*,*,#13528,.F.);
#17592=ORIENTED_EDGE('',*,*,#13529,.F.);
#17593=ORIENTED_EDGE('',*,*,#13530,.T.);
#17594=ORIENTED_EDGE('',*,*,#13531,.T.);
#17595=ORIENTED_EDGE('',*,*,#13532,.F.);
#17596=ORIENTED_EDGE('',*,*,#13533,.T.);
#17597=ORIENTED_EDGE('',*,*,#13534,.T.);
#17598=ORIENTED_EDGE('',*,*,#13535,.T.);
#17599=ORIENTED_EDGE('',*,*,#13536,.T.);
#17600=ORIENTED_EDGE('',*,*,#13537,.T.);
#17601=ORIENTED_EDGE('',*,*,#13538,.T.);
#17602=ORIENTED_EDGE('',*,*,#13539,.T.);
#17603=ORIENTED_EDGE('',*,*,#13540,.F.);
#17604=ORIENTED_EDGE('',*,*,#13541,.T.);
#17605=ORIENTED_EDGE('',*,*,#13542,.T.);
#17606=ORIENTED_EDGE('',*,*,#13543,.T.);
#17607=ORIENTED_EDGE('',*,*,#13544,.T.);
#17608=ORIENTED_EDGE('',*,*,#13545,.T.);
#17609=ORIENTED_EDGE('',*,*,#13546,.T.);
#17610=ORIENTED_EDGE('',*,*,#13547,.T.);
#17611=ORIENTED_EDGE('',*,*,#13548,.T.);
#17612=ORIENTED_EDGE('',*,*,#13549,.T.);
#17613=ORIENTED_EDGE('',*,*,#13462,.F.);
#17614=ORIENTED_EDGE('',*,*,#13550,.T.);
#17615=ORIENTED_EDGE('',*,*,#13551,.T.);
#17616=ORIENTED_EDGE('',*,*,#13457,.T.);
#17617=ORIENTED_EDGE('',*,*,#13552,.F.);
#17618=ORIENTED_EDGE('',*,*,#13507,.F.);
#17619=ORIENTED_EDGE('',*,*,#13508,.F.);
#17620=ORIENTED_EDGE('',*,*,#13464,.T.);
#17621=ORIENTED_EDGE('',*,*,#13553,.F.);
#17622=ORIENTED_EDGE('',*,*,#13554,.F.);
#17623=ORIENTED_EDGE('',*,*,#13555,.T.);
#17624=ORIENTED_EDGE('',*,*,#13556,.F.);
#17625=ORIENTED_EDGE('',*,*,#13557,.T.);
#17626=ORIENTED_EDGE('',*,*,#13558,.F.);
#17627=ORIENTED_EDGE('',*,*,#13559,.T.);
#17628=ORIENTED_EDGE('',*,*,#13560,.F.);
#17629=ORIENTED_EDGE('',*,*,#13561,.T.);
#17630=ORIENTED_EDGE('',*,*,#13562,.T.);
#17631=ORIENTED_EDGE('',*,*,#13563,.T.);
#17632=ORIENTED_EDGE('',*,*,#13564,.F.);
#17633=ORIENTED_EDGE('',*,*,#13565,.T.);
#17634=ORIENTED_EDGE('',*,*,#13566,.F.);
#17635=ORIENTED_EDGE('',*,*,#13567,.T.);
#17636=ORIENTED_EDGE('',*,*,#13568,.F.);
#17637=ORIENTED_EDGE('',*,*,#13569,.T.);
#17638=ORIENTED_EDGE('',*,*,#13570,.T.);
#17639=ORIENTED_EDGE('',*,*,#13571,.T.);
#17640=ORIENTED_EDGE('',*,*,#13572,.F.);
#17641=ORIENTED_EDGE('',*,*,#13573,.T.);
#17642=ORIENTED_EDGE('',*,*,#13574,.T.);
#17643=ORIENTED_EDGE('',*,*,#13575,.T.);
#17644=ORIENTED_EDGE('',*,*,#13576,.F.);
#17645=ORIENTED_EDGE('',*,*,#13577,.T.);
#17646=ORIENTED_EDGE('',*,*,#13578,.T.);
#17647=ORIENTED_EDGE('',*,*,#13579,.T.);
#17648=ORIENTED_EDGE('',*,*,#13580,.T.);
#17649=ORIENTED_EDGE('',*,*,#13581,.T.);
#17650=ORIENTED_EDGE('',*,*,#13582,.T.);
#17651=ORIENTED_EDGE('',*,*,#13583,.T.);
#17652=ORIENTED_EDGE('',*,*,#13584,.F.);
#17653=ORIENTED_EDGE('',*,*,#13585,.T.);
#17654=ORIENTED_EDGE('',*,*,#13586,.T.);
#17655=ORIENTED_EDGE('',*,*,#13587,.T.);
#17656=ORIENTED_EDGE('',*,*,#13588,.T.);
#17657=ORIENTED_EDGE('',*,*,#13589,.T.);
#17658=ORIENTED_EDGE('',*,*,#13590,.T.);
#17659=ORIENTED_EDGE('',*,*,#13591,.T.);
#17660=ORIENTED_EDGE('',*,*,#13592,.T.);
#17661=ORIENTED_EDGE('',*,*,#13593,.T.);
#17662=ORIENTED_EDGE('',*,*,#13560,.T.);
#17663=ORIENTED_EDGE('',*,*,#13594,.T.);
#17664=ORIENTED_EDGE('',*,*,#13542,.F.);
#17665=ORIENTED_EDGE('',*,*,#13595,.T.);
#17666=ORIENTED_EDGE('',*,*,#13538,.F.);
#17667=ORIENTED_EDGE('',*,*,#13596,.T.);
#17668=ORIENTED_EDGE('',*,*,#13564,.T.);
#17669=ORIENTED_EDGE('',*,*,#13597,.T.);
#17670=ORIENTED_EDGE('',*,*,#13534,.F.);
#17671=ORIENTED_EDGE('',*,*,#13598,.T.);
#17672=ORIENTED_EDGE('',*,*,#13568,.T.);
#17673=ORIENTED_EDGE('',*,*,#13599,.T.);
#17674=ORIENTED_EDGE('',*,*,#13572,.T.);
#17675=ORIENTED_EDGE('',*,*,#13600,.T.);
#17676=ORIENTED_EDGE('',*,*,#13530,.F.);
#17677=ORIENTED_EDGE('',*,*,#13601,.T.);
#17678=ORIENTED_EDGE('',*,*,#13516,.T.);
#17679=ORIENTED_EDGE('',*,*,#13602,.T.);
#17680=ORIENTED_EDGE('',*,*,#13586,.F.);
#17681=ORIENTED_EDGE('',*,*,#13603,.T.);
#17682=ORIENTED_EDGE('',*,*,#13578,.F.);
#17683=ORIENTED_EDGE('',*,*,#13604,.T.);
#17684=ORIENTED_EDGE('',*,*,#13524,.T.);
#17685=ORIENTED_EDGE('',*,*,#13605,.T.);
#17686=ORIENTED_EDGE('',*,*,#13573,.F.);
#17687=ORIENTED_EDGE('',*,*,#13601,.F.);
#17688=ORIENTED_EDGE('',*,*,#13529,.T.);
#17689=ORIENTED_EDGE('',*,*,#13606,.T.);
#17690=ORIENTED_EDGE('',*,*,#13229,.F.);
#17691=ORIENTED_EDGE('',*,*,#13243,.F.);
#17692=ORIENTED_EDGE('',*,*,#13257,.F.);
#17693=ORIENTED_EDGE('',*,*,#13271,.F.);
#17694=ORIENTED_EDGE('',*,*,#13285,.F.);
#17695=ORIENTED_EDGE('',*,*,#13299,.F.);
#17696=ORIENTED_EDGE('',*,*,#13313,.F.);
#17697=ORIENTED_EDGE('',*,*,#13327,.F.);
#17698=ORIENTED_EDGE('',*,*,#13341,.F.);
#17699=ORIENTED_EDGE('',*,*,#13355,.F.);
#17700=ORIENTED_EDGE('',*,*,#13369,.F.);
#17701=ORIENTED_EDGE('',*,*,#13383,.F.);
#17702=ORIENTED_EDGE('',*,*,#13397,.F.);
#17703=ORIENTED_EDGE('',*,*,#13411,.F.);
#17704=ORIENTED_EDGE('',*,*,#13425,.F.);
#17705=ORIENTED_EDGE('',*,*,#13593,.F.);
#17706=ORIENTED_EDGE('',*,*,#13607,.F.);
#17707=ORIENTED_EDGE('',*,*,#13509,.T.);
#17708=ORIENTED_EDGE('',*,*,#13458,.T.);
#17709=ORIENTED_EDGE('',*,*,#13592,.F.);
#17710=ORIENTED_EDGE('',*,*,#13608,.T.);
#17711=ORIENTED_EDGE('',*,*,#13510,.T.);
#17712=ORIENTED_EDGE('',*,*,#13607,.T.);
#17713=ORIENTED_EDGE('',*,*,#13512,.T.);
#17714=ORIENTED_EDGE('',*,*,#13609,.T.);
#17715=ORIENTED_EDGE('',*,*,#13590,.F.);
#17716=ORIENTED_EDGE('',*,*,#13610,.T.);
#17717=ORIENTED_EDGE('',*,*,#13514,.T.);
#17718=ORIENTED_EDGE('',*,*,#13611,.T.);
#17719=ORIENTED_EDGE('',*,*,#13588,.F.);
#17720=ORIENTED_EDGE('',*,*,#13612,.T.);
#17721=ORIENTED_EDGE('',*,*,#13582,.F.);
#17722=ORIENTED_EDGE('',*,*,#13613,.T.);
#17723=ORIENTED_EDGE('',*,*,#13520,.T.);
#17724=ORIENTED_EDGE('',*,*,#13614,.T.);
#17725=ORIENTED_EDGE('',*,*,#13580,.F.);
#17726=ORIENTED_EDGE('',*,*,#13615,.T.);
#17727=ORIENTED_EDGE('',*,*,#13522,.T.);
#17728=ORIENTED_EDGE('',*,*,#13616,.T.);
#17729=ORIENTED_EDGE('',*,*,#13528,.T.);
#17730=ORIENTED_EDGE('',*,*,#13617,.T.);
#17731=ORIENTED_EDGE('',*,*,#13574,.F.);
#17732=ORIENTED_EDGE('',*,*,#13606,.F.);
#17733=ORIENTED_EDGE('',*,*,#13526,.F.);
#17734=ORIENTED_EDGE('',*,*,#13618,.T.);
#17735=ORIENTED_EDGE('',*,*,#13576,.T.);
#17736=ORIENTED_EDGE('',*,*,#13619,.T.);
#17737=ORIENTED_EDGE('',*,*,#13584,.T.);
#17738=ORIENTED_EDGE('',*,*,#13620,.T.);
#17739=ORIENTED_EDGE('',*,*,#13518,.F.);
#17740=ORIENTED_EDGE('',*,*,#13621,.T.);
#17741=ORIENTED_EDGE('',*,*,#13525,.F.);
#17742=ORIENTED_EDGE('',*,*,#13604,.F.);
#17743=ORIENTED_EDGE('',*,*,#13577,.F.);
#17744=ORIENTED_EDGE('',*,*,#13618,.F.);
#17745=ORIENTED_EDGE('',*,*,#13523,.F.);
#17746=ORIENTED_EDGE('',*,*,#13615,.F.);
#17747=ORIENTED_EDGE('',*,*,#13579,.F.);
#17748=ORIENTED_EDGE('',*,*,#13605,.F.);
#17749=ORIENTED_EDGE('',*,*,#13521,.F.);
#17750=ORIENTED_EDGE('',*,*,#13613,.F.);
#17751=ORIENTED_EDGE('',*,*,#13581,.F.);
#17752=ORIENTED_EDGE('',*,*,#13616,.F.);
#17753=ORIENTED_EDGE('',*,*,#13583,.F.);
#17754=ORIENTED_EDGE('',*,*,#13614,.F.);
#17755=ORIENTED_EDGE('',*,*,#13519,.F.);
#17756=ORIENTED_EDGE('',*,*,#13620,.F.);
#17757=ORIENTED_EDGE('',*,*,#13513,.F.);
#17758=ORIENTED_EDGE('',*,*,#13610,.F.);
#17759=ORIENTED_EDGE('',*,*,#13589,.F.);
#17760=ORIENTED_EDGE('',*,*,#13611,.F.);
#17761=ORIENTED_EDGE('',*,*,#13515,.F.);
#17762=ORIENTED_EDGE('',*,*,#13612,.F.);
#17763=ORIENTED_EDGE('',*,*,#13587,.F.);
#17764=ORIENTED_EDGE('',*,*,#13602,.F.);
#17765=ORIENTED_EDGE('',*,*,#13517,.F.);
#17766=ORIENTED_EDGE('',*,*,#13603,.F.);
#17767=ORIENTED_EDGE('',*,*,#13585,.F.);
#17768=ORIENTED_EDGE('',*,*,#13621,.F.);
#17769=ORIENTED_EDGE('',*,*,#13575,.F.);
#17770=ORIENTED_EDGE('',*,*,#13617,.F.);
#17771=ORIENTED_EDGE('',*,*,#13527,.F.);
#17772=ORIENTED_EDGE('',*,*,#13619,.F.);
#17773=ORIENTED_EDGE('',*,*,#13511,.F.);
#17774=ORIENTED_EDGE('',*,*,#13608,.F.);
#17775=ORIENTED_EDGE('',*,*,#13591,.F.);
#17776=ORIENTED_EDGE('',*,*,#13609,.F.);
#17777=ORIENTED_EDGE('',*,*,#13536,.F.);
#17778=ORIENTED_EDGE('',*,*,#13622,.T.);
#17779=ORIENTED_EDGE('',*,*,#13566,.T.);
#17780=ORIENTED_EDGE('',*,*,#13623,.T.);
#17781=ORIENTED_EDGE('',*,*,#13558,.T.);
#17782=ORIENTED_EDGE('',*,*,#13624,.T.);
#17783=ORIENTED_EDGE('',*,*,#13544,.F.);
#17784=ORIENTED_EDGE('',*,*,#13625,.T.);
#17785=ORIENTED_EDGE('',*,*,#13556,.T.);
#17786=ORIENTED_EDGE('',*,*,#13626,.T.);
#17787=ORIENTED_EDGE('',*,*,#13546,.F.);
#17788=ORIENTED_EDGE('',*,*,#13627,.T.);
#17789=ORIENTED_EDGE('',*,*,#13548,.F.);
#17790=ORIENTED_EDGE('',*,*,#13628,.T.);
#17791=ORIENTED_EDGE('',*,*,#13554,.T.);
#17792=ORIENTED_EDGE('',*,*,#13629,.F.);
#17793=ORIENTED_EDGE('',*,*,#13553,.T.);
#17794=ORIENTED_EDGE('',*,*,#13463,.F.);
#17795=ORIENTED_EDGE('',*,*,#13549,.F.);
#17796=ORIENTED_EDGE('',*,*,#13629,.T.);
#17797=ORIENTED_EDGE('',*,*,#13570,.F.);
#17798=ORIENTED_EDGE('',*,*,#13630,.T.);
#17799=ORIENTED_EDGE('',*,*,#13532,.T.);
#17800=ORIENTED_EDGE('',*,*,#13631,.T.);
#17801=ORIENTED_EDGE('',*,*,#13540,.T.);
#17802=ORIENTED_EDGE('',*,*,#13632,.T.);
#17803=ORIENTED_EDGE('',*,*,#13562,.F.);
#17804=ORIENTED_EDGE('',*,*,#13633,.T.);
#17805=ORIENTED_EDGE('',*,*,#13569,.F.);
#17806=ORIENTED_EDGE('',*,*,#13598,.F.);
#17807=ORIENTED_EDGE('',*,*,#13533,.F.);
#17808=ORIENTED_EDGE('',*,*,#13630,.F.);
#17809=ORIENTED_EDGE('',*,*,#13535,.F.);
#17810=ORIENTED_EDGE('',*,*,#13599,.F.);
#17811=ORIENTED_EDGE('',*,*,#13567,.F.);
#17812=ORIENTED_EDGE('',*,*,#13622,.F.);
#17813=ORIENTED_EDGE('',*,*,#13537,.F.);
#17814=ORIENTED_EDGE('',*,*,#13623,.F.);
#17815=ORIENTED_EDGE('',*,*,#13565,.F.);
#17816=ORIENTED_EDGE('',*,*,#13596,.F.);
#17817=ORIENTED_EDGE('',*,*,#13539,.F.);
#17818=ORIENTED_EDGE('',*,*,#13597,.F.);
#17819=ORIENTED_EDGE('',*,*,#13563,.F.);
#17820=ORIENTED_EDGE('',*,*,#13632,.F.);
#17821=ORIENTED_EDGE('',*,*,#13545,.F.);
#17822=ORIENTED_EDGE('',*,*,#13624,.F.);
#17823=ORIENTED_EDGE('',*,*,#13557,.F.);
#17824=ORIENTED_EDGE('',*,*,#13627,.F.);
#17825=ORIENTED_EDGE('',*,*,#13543,.F.);
#17826=ORIENTED_EDGE('',*,*,#13594,.F.);
#17827=ORIENTED_EDGE('',*,*,#13559,.F.);
#17828=ORIENTED_EDGE('',*,*,#13625,.F.);
#17829=ORIENTED_EDGE('',*,*,#13561,.F.);
#17830=ORIENTED_EDGE('',*,*,#13595,.F.);
#17831=ORIENTED_EDGE('',*,*,#13541,.F.);
#17832=ORIENTED_EDGE('',*,*,#13633,.F.);
#17833=ORIENTED_EDGE('',*,*,#13531,.F.);
#17834=ORIENTED_EDGE('',*,*,#13600,.F.);
#17835=ORIENTED_EDGE('',*,*,#13571,.F.);
#17836=ORIENTED_EDGE('',*,*,#13631,.F.);
#17837=ORIENTED_EDGE('',*,*,#13547,.F.);
#17838=ORIENTED_EDGE('',*,*,#13626,.F.);
#17839=ORIENTED_EDGE('',*,*,#13555,.F.);
#17840=ORIENTED_EDGE('',*,*,#13628,.F.);
#17841=ORIENTED_EDGE('',*,*,#13456,.F.);
#17842=ORIENTED_EDGE('',*,*,#13427,.T.);
#17843=ORIENTED_EDGE('',*,*,#13505,.T.);
#17844=ORIENTED_EDGE('',*,*,#13552,.T.);
#17845=ORIENTED_EDGE('',*,*,#13634,.T.);
#17846=ORIENTED_EDGE('',*,*,#13237,.T.);
#17847=ORIENTED_EDGE('',*,*,#13234,.T.);
#17848=ORIENTED_EDGE('',*,*,#13437,.F.);
#17849=ORIENTED_EDGE('',*,*,#13551,.F.);
#17850=ORIENTED_EDGE('',*,*,#13461,.T.);
#17851=ORIENTED_EDGE('',*,*,#13238,.T.);
#17852=ORIENTED_EDGE('',*,*,#13634,.F.);
#17853=ORIENTED_EDGE('',*,*,#13550,.F.);
#17854=ORIENTED_EDGE('',*,*,#13423,.T.);
#17855=ORIENTED_EDGE('',*,*,#13432,.F.);
#17856=ORIENTED_EDGE('',*,*,#13409,.T.);
#17857=ORIENTED_EDGE('',*,*,#13418,.F.);
#17858=ORIENTED_EDGE('',*,*,#13395,.T.);
#17859=ORIENTED_EDGE('',*,*,#13404,.F.);
#17860=ORIENTED_EDGE('',*,*,#13381,.T.);
#17861=ORIENTED_EDGE('',*,*,#13390,.F.);
#17862=ORIENTED_EDGE('',*,*,#13367,.T.);
#17863=ORIENTED_EDGE('',*,*,#13376,.F.);
#17864=ORIENTED_EDGE('',*,*,#13353,.T.);
#17865=ORIENTED_EDGE('',*,*,#13362,.F.);
#17866=ORIENTED_EDGE('',*,*,#13339,.T.);
#17867=ORIENTED_EDGE('',*,*,#13348,.F.);
#17868=ORIENTED_EDGE('',*,*,#13325,.T.);
#17869=ORIENTED_EDGE('',*,*,#13334,.F.);
#17870=ORIENTED_EDGE('',*,*,#13311,.T.);
#17871=ORIENTED_EDGE('',*,*,#13320,.F.);
#17872=ORIENTED_EDGE('',*,*,#13297,.T.);
#17873=ORIENTED_EDGE('',*,*,#13306,.F.);
#17874=ORIENTED_EDGE('',*,*,#13283,.T.);
#17875=ORIENTED_EDGE('',*,*,#13292,.F.);
#17876=ORIENTED_EDGE('',*,*,#13269,.T.);
#17877=ORIENTED_EDGE('',*,*,#13278,.F.);
#17878=ORIENTED_EDGE('',*,*,#13255,.T.);
#17879=ORIENTED_EDGE('',*,*,#13264,.F.);
#17880=ORIENTED_EDGE('',*,*,#13241,.T.);
#17881=ORIENTED_EDGE('',*,*,#13250,.F.);
#17882=ORIENTED_EDGE('',*,*,#13227,.T.);
#17883=ORIENTED_EDGE('',*,*,#13236,.F.);
#23843=CYLINDRICAL_SURFACE('',#26230,5.49999999999995);
#23844=CYLINDRICAL_SURFACE('',#26233,3.49999999999995);
#23845=CYLINDRICAL_SURFACE('',#26244,5.49999999999995);
#23846=CYLINDRICAL_SURFACE('',#26247,3.49999999999995);
#23847=CYLINDRICAL_SURFACE('',#26258,5.49999999999995);
#23848=CYLINDRICAL_SURFACE('',#26261,3.49999999999995);
#23849=CYLINDRICAL_SURFACE('',#26272,5.49999999999995);
#23850=CYLINDRICAL_SURFACE('',#26275,3.49999999999995);
#23851=CYLINDRICAL_SURFACE('',#26286,5.49999999999995);
#23852=CYLINDRICAL_SURFACE('',#26289,3.49999999999995);
#23853=CYLINDRICAL_SURFACE('',#26300,5.49999999999995);
#23854=CYLINDRICAL_SURFACE('',#26303,3.49999999999995);
#23855=CYLINDRICAL_SURFACE('',#26314,5.50000000000001);
#23856=CYLINDRICAL_SURFACE('',#26317,3.5);
#23857=CYLINDRICAL_SURFACE('',#26328,5.50000000000001);
#23858=CYLINDRICAL_SURFACE('',#26331,3.5);
#23859=CYLINDRICAL_SURFACE('',#26342,5.50000000000001);
#23860=CYLINDRICAL_SURFACE('',#26345,3.5);
#23861=CYLINDRICAL_SURFACE('',#26356,5.50000000000001);
#23862=CYLINDRICAL_SURFACE('',#26359,3.5);
#23863=CYLINDRICAL_SURFACE('',#26370,5.50000000000001);
#23864=CYLINDRICAL_SURFACE('',#26373,3.5);
#23865=CYLINDRICAL_SURFACE('',#26384,5.50000000000001);
#23866=CYLINDRICAL_SURFACE('',#26387,3.5);
#23867=CYLINDRICAL_SURFACE('',#26398,5.50000000000001);
#23868=CYLINDRICAL_SURFACE('',#26401,3.5);
#23869=CYLINDRICAL_SURFACE('',#26412,5.5);
#23870=CYLINDRICAL_SURFACE('',#26415,3.5);
#23871=CYLINDRICAL_SURFACE('',#26426,5.5);
#23872=CYLINDRICAL_SURFACE('',#26429,3.5);
#23873=CYLINDRICAL_SURFACE('',#26547,2.3);
#23874=CYLINDRICAL_SURFACE('',#26548,2.3);
#23875=CYLINDRICAL_SURFACE('',#26549,0.5);
#23876=CYLINDRICAL_SURFACE('',#26550,0.5);
#23877=CYLINDRICAL_SURFACE('',#26551,0.5);
#23878=CYLINDRICAL_SURFACE('',#26552,0.5);
#23879=CYLINDRICAL_SURFACE('',#26553,0.5);
#23880=CYLINDRICAL_SURFACE('',#26554,0.5);
#23881=CYLINDRICAL_SURFACE('',#26555,0.5);
#23882=CYLINDRICAL_SURFACE('',#26556,0.5);
#23883=CYLINDRICAL_SURFACE('',#26557,1.);
#23884=CYLINDRICAL_SURFACE('',#26563,2.3);
#23885=CYLINDRICAL_SURFACE('',#26564,2.3);
#23886=CYLINDRICAL_SURFACE('',#26565,0.5);
#23887=CYLINDRICAL_SURFACE('',#26566,0.5);
#23888=CYLINDRICAL_SURFACE('',#26567,0.5);
#23889=CYLINDRICAL_SURFACE('',#26568,0.5);
#23890=CYLINDRICAL_SURFACE('',#26569,0.5);
#23891=CYLINDRICAL_SURFACE('',#26570,0.5);
#23892=CYLINDRICAL_SURFACE('',#26571,0.5);
#23893=CYLINDRICAL_SURFACE('',#26572,0.5);
#23894=CYLINDRICAL_SURFACE('',#26573,1.);
#24316=ADVANCED_FACE('',(#2363),#23843,.F.);
#24317=ADVANCED_FACE('',(#2364),#23844,.F.);
#24318=ADVANCED_FACE('',(#2365),#23845,.F.);
#24319=ADVANCED_FACE('',(#2366),#23846,.F.);
#24320=ADVANCED_FACE('',(#2367),#23847,.F.);
#24321=ADVANCED_FACE('',(#2368),#23848,.F.);
#24322=ADVANCED_FACE('',(#2369),#23849,.F.);
#24323=ADVANCED_FACE('',(#2370),#23850,.F.);
#24324=ADVANCED_FACE('',(#2371),#23851,.F.);
#24325=ADVANCED_FACE('',(#2372),#23852,.F.);
#24326=ADVANCED_FACE('',(#2373),#23853,.F.);
#24327=ADVANCED_FACE('',(#2374),#23854,.F.);
#24328=ADVANCED_FACE('',(#2375),#23855,.F.);
#24329=ADVANCED_FACE('',(#2376),#23856,.F.);
#24330=ADVANCED_FACE('',(#2377),#23857,.F.);
#24331=ADVANCED_FACE('',(#2378),#23858,.F.);
#24332=ADVANCED_FACE('',(#2379),#23859,.F.);
#24333=ADVANCED_FACE('',(#2380),#23860,.F.);
#24334=ADVANCED_FACE('',(#2381),#23861,.F.);
#24335=ADVANCED_FACE('',(#2382),#23862,.F.);
#24336=ADVANCED_FACE('',(#2383),#23863,.F.);
#24337=ADVANCED_FACE('',(#2384),#23864,.F.);
#24338=ADVANCED_FACE('',(#2385),#23865,.F.);
#24339=ADVANCED_FACE('',(#2386),#23866,.F.);
#24340=ADVANCED_FACE('',(#2387),#23867,.F.);
#24341=ADVANCED_FACE('',(#2388),#23868,.F.);
#24342=ADVANCED_FACE('',(#2389),#23869,.F.);
#24343=ADVANCED_FACE('',(#2390),#23870,.F.);
#24344=ADVANCED_FACE('',(#2391),#23871,.F.);
#24345=ADVANCED_FACE('',(#2392),#23872,.F.);
#24346=ADVANCED_FACE('',(#2393),#1551,.F.);
#24347=ADVANCED_FACE('',(#2394),#1552,.F.);
#24348=ADVANCED_FACE('',(#2395),#1553,.T.);
#24349=ADVANCED_FACE('',(#2396),#1554,.F.);
#24350=ADVANCED_FACE('',(#2397),#1555,.T.);
#24351=ADVANCED_FACE('',(#2398),#1556,.F.);
#24352=ADVANCED_FACE('',(#2399),#1557,.F.);
#24353=ADVANCED_FACE('',(#2400),#1558,.F.);
#24354=ADVANCED_FACE('',(#2401),#1559,.F.);
#24355=ADVANCED_FACE('',(#2402),#1560,.F.);
#24356=ADVANCED_FACE('',(#2403),#1561,.F.);
#24357=ADVANCED_FACE('',(#2404),#1562,.F.);
#24358=ADVANCED_FACE('',(#2405),#1563,.F.);
#24359=ADVANCED_FACE('',(#2406),#1564,.F.);
#24360=ADVANCED_FACE('',(#2407),#1565,.F.);
#24361=ADVANCED_FACE('',(#2408),#1566,.F.);
#24362=ADVANCED_FACE('',(#2409),#1567,.F.);
#24363=ADVANCED_FACE('',(#2410),#1568,.F.);
#24364=ADVANCED_FACE('',(#2411),#1569,.F.);
#24365=ADVANCED_FACE('',(#2412),#1570,.F.);
#24366=ADVANCED_FACE('',(#2413),#1571,.F.);
#24367=ADVANCED_FACE('',(#2414),#1572,.F.);
#24368=ADVANCED_FACE('',(#2415),#1573,.F.);
#24369=ADVANCED_FACE('',(#2416),#1574,.F.);
#24370=ADVANCED_FACE('',(#2417),#1575,.F.);
#24371=ADVANCED_FACE('',(#2418),#1576,.F.);
#24372=ADVANCED_FACE('',(#2419),#1577,.F.);
#24373=ADVANCED_FACE('',(#2420),#1578,.F.);
#24374=ADVANCED_FACE('',(#2421),#1579,.F.);
#24375=ADVANCED_FACE('',(#2422),#1580,.F.);
#24376=ADVANCED_FACE('',(#2423),#1581,.F.);
#24377=ADVANCED_FACE('',(#2424),#1582,.F.);
#24378=ADVANCED_FACE('',(#2425),#1583,.F.);
#24379=ADVANCED_FACE('',(#2426),#1584,.F.);
#24380=ADVANCED_FACE('',(#2427),#1585,.F.);
#24381=ADVANCED_FACE('',(#2428),#1586,.F.);
#24382=ADVANCED_FACE('',(#2429),#1587,.F.);
#24383=ADVANCED_FACE('',(#2430),#1588,.F.);
#24384=ADVANCED_FACE('',(#2431),#1589,.F.);
#24385=ADVANCED_FACE('',(#2432),#1590,.F.);
#24386=ADVANCED_FACE('',(#2433),#1591,.F.);
#24387=ADVANCED_FACE('',(#2434),#1592,.F.);
#24388=ADVANCED_FACE('',(#2435),#1593,.F.);
#24389=ADVANCED_FACE('',(#2436),#1594,.F.);
#24390=ADVANCED_FACE('',(#2437),#1595,.F.);
#24391=ADVANCED_FACE('',(#2438),#1596,.F.);
#24392=ADVANCED_FACE('',(#2439),#1597,.F.);
#24393=ADVANCED_FACE('',(#2440),#1598,.T.);
#24394=ADVANCED_FACE('',(#2441),#1599,.F.);
#24395=ADVANCED_FACE('',(#2442),#1600,.F.);
#24396=ADVANCED_FACE('',(#2443),#1601,.F.);
#24397=ADVANCED_FACE('',(#2444),#1602,.F.);
#24398=ADVANCED_FACE('',(#2445),#1603,.F.);
#24399=ADVANCED_FACE('',(#2446),#1604,.T.);
#24400=ADVANCED_FACE('',(#2447),#1605,.T.);
#24401=ADVANCED_FACE('',(#2448,#1247,#1248,#1249,#1250,#1251,#1252,#1253,
#1254,#1255,#1256,#1257,#1258,#1259,#1260,#1261),#1606,.T.);
#24402=ADVANCED_FACE('',(#2449),#1607,.T.);
#24403=ADVANCED_FACE('',(#2450),#1608,.T.);
#24404=ADVANCED_FACE('',(#2451),#1609,.T.);
#24405=ADVANCED_FACE('',(#2452),#1610,.T.);
#24406=ADVANCED_FACE('',(#2453),#1611,.T.);
#24407=ADVANCED_FACE('',(#2454),#1612,.T.);
#24408=ADVANCED_FACE('',(#2455),#1613,.T.);
#24409=ADVANCED_FACE('',(#2456),#23873,.F.);
#24410=ADVANCED_FACE('',(#2457),#23874,.F.);
#24411=ADVANCED_FACE('',(#2458),#23875,.T.);
#24412=ADVANCED_FACE('',(#2459),#23876,.T.);
#24413=ADVANCED_FACE('',(#2460),#23877,.T.);
#24414=ADVANCED_FACE('',(#2461),#23878,.T.);
#24415=ADVANCED_FACE('',(#2462),#23879,.F.);
#24416=ADVANCED_FACE('',(#2463),#23880,.F.);
#24417=ADVANCED_FACE('',(#2464),#23881,.T.);
#24418=ADVANCED_FACE('',(#2465),#23882,.T.);
#24419=ADVANCED_FACE('',(#2466),#23883,.T.);
#24420=ADVANCED_FACE('',(#2467),#1614,.F.);
#24421=ADVANCED_FACE('',(#2468),#1615,.F.);
#24422=ADVANCED_FACE('',(#2469),#1616,.F.);
#24423=ADVANCED_FACE('',(#2470),#1617,.F.);
#24424=ADVANCED_FACE('',(#2471),#1618,.F.);
#24425=ADVANCED_FACE('',(#2472),#23884,.F.);
#24426=ADVANCED_FACE('',(#2473),#23885,.F.);
#24427=ADVANCED_FACE('',(#2474),#23886,.T.);
#24428=ADVANCED_FACE('',(#2475),#23887,.T.);
#24429=ADVANCED_FACE('',(#2476),#23888,.T.);
#24430=ADVANCED_FACE('',(#2477),#23889,.T.);
#24431=ADVANCED_FACE('',(#2478),#23890,.F.);
#24432=ADVANCED_FACE('',(#2479),#23891,.F.);
#24433=ADVANCED_FACE('',(#2480),#23892,.T.);
#24434=ADVANCED_FACE('',(#2481),#23893,.T.);
#24435=ADVANCED_FACE('',(#2482),#23894,.T.);
#24436=ADVANCED_FACE('',(#2483),#1619,.F.);
#24437=ADVANCED_FACE('',(#2484),#1620,.F.);
#24438=ADVANCED_FACE('',(#2485),#1621,.F.);
#24439=ADVANCED_FACE('',(#2486,#1262),#1622,.F.);
#24440=ADVANCED_FACE('',(#2487,#1263),#1623,.F.);
#24441=ADVANCED_FACE('',(#2488,#1264),#1624,.F.);
#24442=ADVANCED_FACE('',(#2489,#1265),#1625,.F.);
#24443=ADVANCED_FACE('',(#2490,#1266),#1626,.F.);
#24444=ADVANCED_FACE('',(#2491,#1267),#1627,.F.);
#24445=ADVANCED_FACE('',(#2492,#1268),#1628,.F.);
#24446=ADVANCED_FACE('',(#2493,#1269),#1629,.F.);
#24447=ADVANCED_FACE('',(#2494,#1270),#1630,.F.);
#24448=ADVANCED_FACE('',(#2495,#1271),#1631,.F.);
#24449=ADVANCED_FACE('',(#2496,#1272),#1632,.F.);
#24450=ADVANCED_FACE('',(#2497,#1273),#1633,.F.);
#24451=ADVANCED_FACE('',(#2498,#1274),#1634,.F.);
#24452=ADVANCED_FACE('',(#2499,#1275),#1635,.F.);
#24453=ADVANCED_FACE('',(#2500,#1276),#1636,.F.);
#25670=CLOSED_SHELL('',(#24316,#24317,#24318,#24319,#24320,#24321,#24322,
#24323,#24324,#24325,#24326,#24327,#24328,#24329,#24330,#24331,#24332,#24333,
#24334,#24335,#24336,#24337,#24338,#24339,#24340,#24341,#24342,#24343,#24344,
#24345,#24346,#24347,#24348,#24349,#24350,#24351,#24352,#24353,#24354,#24355,
#24356,#24357,#24358,#24359,#24360,#24361,#24362,#24363,#24364,#24365,#24366,
#24367,#24368,#24369,#24370,#24371,#24372,#24373,#24374,#24375,#24376,#24377,
#24378,#24379,#24380,#24381,#24382,#24383,#24384,#24385,#24386,#24387,#24388,
#24389,#24390,#24391,#24392,#24393,#24394,#24395,#24396,#24397,#24398,#24399,
#24400,#24401,#24402,#24403,#24404,#24405,#24406,#24407,#24408,#24409,#24410,
#24411,#24412,#24413,#24414,#24415,#24416,#24417,#24418,#24419,#24420,#24421,
#24422,#24423,#24424,#24425,#24426,#24427,#24428,#24429,#24430,#24431,#24432,
#24433,#24434,#24435,#24436,#24437,#24438,#24439,#24440,#24441,#24442,#24443,
#24444,#24445,#24446,#24447,#24448,#24449,#24450,#24451,#24452,#24453));
#26229=AXIS2_PLACEMENT_3D('',#36676,#29287,#29288);
#26230=AXIS2_PLACEMENT_3D('',#36677,#29289,#29290);
#26231=AXIS2_PLACEMENT_3D('',#36679,#29291,#29292);
#26232=AXIS2_PLACEMENT_3D('',#36682,#29294,#29295);
#26233=AXIS2_PLACEMENT_3D('',#36683,#29296,#29297);
#26234=AXIS2_PLACEMENT_3D('',#36686,#29298,#29299);
#26235=AXIS2_PLACEMENT_3D('',#36688,#29300,#29301);
#26236=AXIS2_PLACEMENT_3D('',#36690,#29302,#29303);
#26237=AXIS2_PLACEMENT_3D('',#36692,#29304,#29305);
#26238=AXIS2_PLACEMENT_3D('',#36694,#29306,#29307);
#26239=AXIS2_PLACEMENT_3D('',#36697,#29309,#29310);
#26240=AXIS2_PLACEMENT_3D('',#36699,#29311,#29312);
#26241=AXIS2_PLACEMENT_3D('',#36701,#29313,#29314);
#26242=AXIS2_PLACEMENT_3D('',#36703,#29315,#29316);
#26243=AXIS2_PLACEMENT_3D('',#36704,#29317,#29318);
#26244=AXIS2_PLACEMENT_3D('',#36705,#29319,#29320);
#26245=AXIS2_PLACEMENT_3D('',#36707,#29321,#29322);
#26246=AXIS2_PLACEMENT_3D('',#36710,#29324,#29325);
#26247=AXIS2_PLACEMENT_3D('',#36711,#29326,#29327);
#26248=AXIS2_PLACEMENT_3D('',#36714,#29328,#29329);
#26249=AXIS2_PLACEMENT_3D('',#36716,#29330,#29331);
#26250=AXIS2_PLACEMENT_3D('',#36718,#29332,#29333);
#26251=AXIS2_PLACEMENT_3D('',#36720,#29334,#29335);
#26252=AXIS2_PLACEMENT_3D('',#36722,#29336,#29337);
#26253=AXIS2_PLACEMENT_3D('',#36725,#29339,#29340);
#26254=AXIS2_PLACEMENT_3D('',#36727,#29341,#29342);
#26255=AXIS2_PLACEMENT_3D('',#36729,#29343,#29344);
#26256=AXIS2_PLACEMENT_3D('',#36731,#29345,#29346);
#26257=AXIS2_PLACEMENT_3D('',#36732,#29347,#29348);
#26258=AXIS2_PLACEMENT_3D('',#36733,#29349,#29350);
#26259=AXIS2_PLACEMENT_3D('',#36735,#29351,#29352);
#26260=AXIS2_PLACEMENT_3D('',#36738,#29354,#29355);
#26261=AXIS2_PLACEMENT_3D('',#36739,#29356,#29357);
#26262=AXIS2_PLACEMENT_3D('',#36742,#29358,#29359);
#26263=AXIS2_PLACEMENT_3D('',#36744,#29360,#29361);
#26264=AXIS2_PLACEMENT_3D('',#36746,#29362,#29363);
#26265=AXIS2_PLACEMENT_3D('',#36748,#29364,#29365);
#26266=AXIS2_PLACEMENT_3D('',#36750,#29366,#29367);
#26267=AXIS2_PLACEMENT_3D('',#36753,#29369,#29370);
#26268=AXIS2_PLACEMENT_3D('',#36755,#29371,#29372);
#26269=AXIS2_PLACEMENT_3D('',#36757,#29373,#29374);
#26270=AXIS2_PLACEMENT_3D('',#36759,#29375,#29376);
#26271=AXIS2_PLACEMENT_3D('',#36760,#29377,#29378);
#26272=AXIS2_PLACEMENT_3D('',#36761,#29379,#29380);
#26273=AXIS2_PLACEMENT_3D('',#36763,#29381,#29382);
#26274=AXIS2_PLACEMENT_3D('',#36766,#29384,#29385);
#26275=AXIS2_PLACEMENT_3D('',#36767,#29386,#29387);
#26276=AXIS2_PLACEMENT_3D('',#36770,#29388,#29389);
#26277=AXIS2_PLACEMENT_3D('',#36772,#29390,#29391);
#26278=AXIS2_PLACEMENT_3D('',#36774,#29392,#29393);
#26279=AXIS2_PLACEMENT_3D('',#36776,#29394,#29395);
#26280=AXIS2_PLACEMENT_3D('',#36778,#29396,#29397);
#26281=AXIS2_PLACEMENT_3D('',#36781,#29399,#29400);
#26282=AXIS2_PLACEMENT_3D('',#36783,#29401,#29402);
#26283=AXIS2_PLACEMENT_3D('',#36785,#29403,#29404);
#26284=AXIS2_PLACEMENT_3D('',#36787,#29405,#29406);
#26285=AXIS2_PLACEMENT_3D('',#36788,#29407,#29408);
#26286=AXIS2_PLACEMENT_3D('',#36789,#29409,#29410);
#26287=AXIS2_PLACEMENT_3D('',#36791,#29411,#29412);
#26288=AXIS2_PLACEMENT_3D('',#36794,#29414,#29415);
#26289=AXIS2_PLACEMENT_3D('',#36795,#29416,#29417);
#26290=AXIS2_PLACEMENT_3D('',#36798,#29418,#29419);
#26291=AXIS2_PLACEMENT_3D('',#36800,#29420,#29421);
#26292=AXIS2_PLACEMENT_3D('',#36802,#29422,#29423);
#26293=AXIS2_PLACEMENT_3D('',#36804,#29424,#29425);
#26294=AXIS2_PLACEMENT_3D('',#36806,#29426,#29427);
#26295=AXIS2_PLACEMENT_3D('',#36809,#29429,#29430);
#26296=AXIS2_PLACEMENT_3D('',#36811,#29431,#29432);
#26297=AXIS2_PLACEMENT_3D('',#36813,#29433,#29434);
#26298=AXIS2_PLACEMENT_3D('',#36815,#29435,#29436);
#26299=AXIS2_PLACEMENT_3D('',#36816,#29437,#29438);
#26300=AXIS2_PLACEMENT_3D('',#36817,#29439,#29440);
#26301=AXIS2_PLACEMENT_3D('',#36819,#29441,#29442);
#26302=AXIS2_PLACEMENT_3D('',#36822,#29444,#29445);
#26303=AXIS2_PLACEMENT_3D('',#36823,#29446,#29447);
#26304=AXIS2_PLACEMENT_3D('',#36826,#29448,#29449);
#26305=AXIS2_PLACEMENT_3D('',#36828,#29450,#29451);
#26306=AXIS2_PLACEMENT_3D('',#36830,#29452,#29453);
#26307=AXIS2_PLACEMENT_3D('',#36832,#29454,#29455);
#26308=AXIS2_PLACEMENT_3D('',#36834,#29456,#29457);
#26309=AXIS2_PLACEMENT_3D('',#36837,#29459,#29460);
#26310=AXIS2_PLACEMENT_3D('',#36839,#29461,#29462);
#26311=AXIS2_PLACEMENT_3D('',#36841,#29463,#29464);
#26312=AXIS2_PLACEMENT_3D('',#36843,#29465,#29466);
#26313=AXIS2_PLACEMENT_3D('',#36844,#29467,#29468);
#26314=AXIS2_PLACEMENT_3D('',#36845,#29469,#29470);
#26315=AXIS2_PLACEMENT_3D('',#36847,#29471,#29472);
#26316=AXIS2_PLACEMENT_3D('',#36850,#29474,#29475);
#26317=AXIS2_PLACEMENT_3D('',#36851,#29476,#29477);
#26318=AXIS2_PLACEMENT_3D('',#36854,#29478,#29479);
#26319=AXIS2_PLACEMENT_3D('',#36856,#29480,#29481);
#26320=AXIS2_PLACEMENT_3D('',#36858,#29482,#29483);
#26321=AXIS2_PLACEMENT_3D('',#36860,#29484,#29485);
#26322=AXIS2_PLACEMENT_3D('',#36862,#29486,#29487);
#26323=AXIS2_PLACEMENT_3D('',#36865,#29489,#29490);
#26324=AXIS2_PLACEMENT_3D('',#36867,#29491,#29492);
#26325=AXIS2_PLACEMENT_3D('',#36869,#29493,#29494);
#26326=AXIS2_PLACEMENT_3D('',#36871,#29495,#29496);
#26327=AXIS2_PLACEMENT_3D('',#36872,#29497,#29498);
#26328=AXIS2_PLACEMENT_3D('',#36873,#29499,#29500);
#26329=AXIS2_PLACEMENT_3D('',#36875,#29501,#29502);
#26330=AXIS2_PLACEMENT_3D('',#36878,#29504,#29505);
#26331=AXIS2_PLACEMENT_3D('',#36879,#29506,#29507);
#26332=AXIS2_PLACEMENT_3D('',#36882,#29508,#29509);
#26333=AXIS2_PLACEMENT_3D('',#36884,#29510,#29511);
#26334=AXIS2_PLACEMENT_3D('',#36886,#29512,#29513);
#26335=AXIS2_PLACEMENT_3D('',#36888,#29514,#29515);
#26336=AXIS2_PLACEMENT_3D('',#36890,#29516,#29517);
#26337=AXIS2_PLACEMENT_3D('',#36893,#29519,#29520);
#26338=AXIS2_PLACEMENT_3D('',#36895,#29521,#29522);
#26339=AXIS2_PLACEMENT_3D('',#36897,#29523,#29524);
#26340=AXIS2_PLACEMENT_3D('',#36899,#29525,#29526);
#26341=AXIS2_PLACEMENT_3D('',#36900,#29527,#29528);
#26342=AXIS2_PLACEMENT_3D('',#36901,#29529,#29530);
#26343=AXIS2_PLACEMENT_3D('',#36903,#29531,#29532);
#26344=AXIS2_PLACEMENT_3D('',#36906,#29534,#29535);
#26345=AXIS2_PLACEMENT_3D('',#36907,#29536,#29537);
#26346=AXIS2_PLACEMENT_3D('',#36910,#29538,#29539);
#26347=AXIS2_PLACEMENT_3D('',#36912,#29540,#29541);
#26348=AXIS2_PLACEMENT_3D('',#36914,#29542,#29543);
#26349=AXIS2_PLACEMENT_3D('',#36916,#29544,#29545);
#26350=AXIS2_PLACEMENT_3D('',#36918,#29546,#29547);
#26351=AXIS2_PLACEMENT_3D('',#36921,#29549,#29550);
#26352=AXIS2_PLACEMENT_3D('',#36923,#29551,#29552);
#26353=AXIS2_PLACEMENT_3D('',#36925,#29553,#29554);
#26354=AXIS2_PLACEMENT_3D('',#36927,#29555,#29556);
#26355=AXIS2_PLACEMENT_3D('',#36928,#29557,#29558);
#26356=AXIS2_PLACEMENT_3D('',#36929,#29559,#29560);
#26357=AXIS2_PLACEMENT_3D('',#36931,#29561,#29562);
#26358=AXIS2_PLACEMENT_3D('',#36934,#29564,#29565);
#26359=AXIS2_PLACEMENT_3D('',#36935,#29566,#29567);
#26360=AXIS2_PLACEMENT_3D('',#36938,#29568,#29569);
#26361=AXIS2_PLACEMENT_3D('',#36940,#29570,#29571);
#26362=AXIS2_PLACEMENT_3D('',#36942,#29572,#29573);
#26363=AXIS2_PLACEMENT_3D('',#36944,#29574,#29575);
#26364=AXIS2_PLACEMENT_3D('',#36946,#29576,#29577);
#26365=AXIS2_PLACEMENT_3D('',#36949,#29579,#29580);
#26366=AXIS2_PLACEMENT_3D('',#36951,#29581,#29582);
#26367=AXIS2_PLACEMENT_3D('',#36953,#29583,#29584);
#26368=AXIS2_PLACEMENT_3D('',#36955,#29585,#29586);
#26369=AXIS2_PLACEMENT_3D('',#36956,#29587,#29588);
#26370=AXIS2_PLACEMENT_3D('',#36957,#29589,#29590);
#26371=AXIS2_PLACEMENT_3D('',#36959,#29591,#29592);
#26372=AXIS2_PLACEMENT_3D('',#36962,#29594,#29595);
#26373=AXIS2_PLACEMENT_3D('',#36963,#29596,#29597);
#26374=AXIS2_PLACEMENT_3D('',#36966,#29598,#29599);
#26375=AXIS2_PLACEMENT_3D('',#36968,#29600,#29601);
#26376=AXIS2_PLACEMENT_3D('',#36970,#29602,#29603);
#26377=AXIS2_PLACEMENT_3D('',#36972,#29604,#29605);
#26378=AXIS2_PLACEMENT_3D('',#36974,#29606,#29607);
#26379=AXIS2_PLACEMENT_3D('',#36977,#29609,#29610);
#26380=AXIS2_PLACEMENT_3D('',#36979,#29611,#29612);
#26381=AXIS2_PLACEMENT_3D('',#36981,#29613,#29614);
#26382=AXIS2_PLACEMENT_3D('',#36983,#29615,#29616);
#26383=AXIS2_PLACEMENT_3D('',#36984,#29617,#29618);
#26384=AXIS2_PLACEMENT_3D('',#36985,#29619,#29620);
#26385=AXIS2_PLACEMENT_3D('',#36987,#29621,#29622);
#26386=AXIS2_PLACEMENT_3D('',#36990,#29624,#29625);
#26387=AXIS2_PLACEMENT_3D('',#36991,#29626,#29627);
#26388=AXIS2_PLACEMENT_3D('',#36994,#29628,#29629);
#26389=AXIS2_PLACEMENT_3D('',#36996,#29630,#29631);
#26390=AXIS2_PLACEMENT_3D('',#36998,#29632,#29633);
#26391=AXIS2_PLACEMENT_3D('',#37000,#29634,#29635);
#26392=AXIS2_PLACEMENT_3D('',#37002,#29636,#29637);
#26393=AXIS2_PLACEMENT_3D('',#37005,#29639,#29640);
#26394=AXIS2_PLACEMENT_3D('',#37007,#29641,#29642);
#26395=AXIS2_PLACEMENT_3D('',#37009,#29643,#29644);
#26396=AXIS2_PLACEMENT_3D('',#37011,#29645,#29646);
#26397=AXIS2_PLACEMENT_3D('',#37012,#29647,#29648);
#26398=AXIS2_PLACEMENT_3D('',#37013,#29649,#29650);
#26399=AXIS2_PLACEMENT_3D('',#37015,#29651,#29652);
#26400=AXIS2_PLACEMENT_3D('',#37018,#29654,#29655);
#26401=AXIS2_PLACEMENT_3D('',#37019,#29656,#29657);
#26402=AXIS2_PLACEMENT_3D('',#37022,#29658,#29659);
#26403=AXIS2_PLACEMENT_3D('',#37024,#29660,#29661);
#26404=AXIS2_PLACEMENT_3D('',#37026,#29662,#29663);
#26405=AXIS2_PLACEMENT_3D('',#37028,#29664,#29665);
#26406=AXIS2_PLACEMENT_3D('',#37030,#29666,#29667);
#26407=AXIS2_PLACEMENT_3D('',#37033,#29669,#29670);
#26408=AXIS2_PLACEMENT_3D('',#37035,#29671,#29672);
#26409=AXIS2_PLACEMENT_3D('',#37037,#29673,#29674);
#26410=AXIS2_PLACEMENT_3D('',#37039,#29675,#29676);
#26411=AXIS2_PLACEMENT_3D('',#37040,#29677,#29678);
#26412=AXIS2_PLACEMENT_3D('',#37041,#29679,#29680);
#26413=AXIS2_PLACEMENT_3D('',#37043,#29681,#29682);
#26414=AXIS2_PLACEMENT_3D('',#37046,#29684,#29685);
#26415=AXIS2_PLACEMENT_3D('',#37047,#29686,#29687);
#26416=AXIS2_PLACEMENT_3D('',#37050,#29688,#29689);
#26417=AXIS2_PLACEMENT_3D('',#37052,#29690,#29691);
#26418=AXIS2_PLACEMENT_3D('',#37054,#29692,#29693);
#26419=AXIS2_PLACEMENT_3D('',#37056,#29694,#29695);
#26420=AXIS2_PLACEMENT_3D('',#37058,#29696,#29697);
#26421=AXIS2_PLACEMENT_3D('',#37061,#29699,#29700);
#26422=AXIS2_PLACEMENT_3D('',#37063,#29701,#29702);
#26423=AXIS2_PLACEMENT_3D('',#37065,#29703,#29704);
#26424=AXIS2_PLACEMENT_3D('',#37067,#29705,#29706);
#26425=AXIS2_PLACEMENT_3D('',#37068,#29707,#29708);
#26426=AXIS2_PLACEMENT_3D('',#37069,#29709,#29710);
#26427=AXIS2_PLACEMENT_3D('',#37071,#29711,#29712);
#26428=AXIS2_PLACEMENT_3D('',#37074,#29714,#29715);
#26429=AXIS2_PLACEMENT_3D('',#37075,#29716,#29717);
#26430=AXIS2_PLACEMENT_3D('',#37078,#29718,#29719);
#26431=AXIS2_PLACEMENT_3D('',#37080,#29720,#29721);
#26432=AXIS2_PLACEMENT_3D('',#37082,#29722,#29723);
#26433=AXIS2_PLACEMENT_3D('',#37084,#29724,#29725);
#26434=AXIS2_PLACEMENT_3D('',#37086,#29726,#29727);
#26435=AXIS2_PLACEMENT_3D('',#37089,#29729,#29730);
#26436=AXIS2_PLACEMENT_3D('',#37091,#29731,#29732);
#26437=AXIS2_PLACEMENT_3D('',#37093,#29733,#29734);
#26438=AXIS2_PLACEMENT_3D('',#37095,#29735,#29736);
#26439=AXIS2_PLACEMENT_3D('',#37096,#29737,#29738);
#26440=AXIS2_PLACEMENT_3D('',#37097,#29739,#29740);
#26441=AXIS2_PLACEMENT_3D('',#37103,#29744,#29745);
#26442=AXIS2_PLACEMENT_3D('',#37106,#29748,#29749);
#26443=AXIS2_PLACEMENT_3D('',#37128,#29768,#29769);
#26444=AXIS2_PLACEMENT_3D('',#37130,#29771,#29772);
#26445=AXIS2_PLACEMENT_3D('',#37153,#29791,#29792);
#26446=AXIS2_PLACEMENT_3D('',#37154,#29793,#29794);
#26447=AXIS2_PLACEMENT_3D('',#37157,#29797,#29798);
#26448=AXIS2_PLACEMENT_3D('',#37158,#29799,#29800);
#26449=AXIS2_PLACEMENT_3D('',#37159,#29801,#29802);
#26450=AXIS2_PLACEMENT_3D('',#37162,#29805,#29806);
#26451=AXIS2_PLACEMENT_3D('',#37163,#29807,#29808);
#26452=AXIS2_PLACEMENT_3D('',#37164,#29809,#29810);
#26453=AXIS2_PLACEMENT_3D('',#37167,#29813,#29814);
#26454=AXIS2_PLACEMENT_3D('',#37168,#29815,#29816);
#26455=AXIS2_PLACEMENT_3D('',#37169,#29817,#29818);
#26456=AXIS2_PLACEMENT_3D('',#37172,#29821,#29822);
#26457=AXIS2_PLACEMENT_3D('',#37173,#29823,#29824);
#26458=AXIS2_PLACEMENT_3D('',#37174,#29825,#29826);
#26459=AXIS2_PLACEMENT_3D('',#37177,#29829,#29830);
#26460=AXIS2_PLACEMENT_3D('',#37178,#29831,#29832);
#26461=AXIS2_PLACEMENT_3D('',#37179,#29833,#29834);
#26462=AXIS2_PLACEMENT_3D('',#37182,#29837,#29838);
#26463=AXIS2_PLACEMENT_3D('',#37183,#29839,#29840);
#26464=AXIS2_PLACEMENT_3D('',#37184,#29841,#29842);
#26465=AXIS2_PLACEMENT_3D('',#37187,#29845,#29846);
#26466=AXIS2_PLACEMENT_3D('',#37188,#29847,#29848);
#26467=AXIS2_PLACEMENT_3D('',#37189,#29849,#29850);
#26468=AXIS2_PLACEMENT_3D('',#37192,#29853,#29854);
#26469=AXIS2_PLACEMENT_3D('',#37193,#29855,#29856);
#26470=AXIS2_PLACEMENT_3D('',#37194,#29857,#29858);
#26471=AXIS2_PLACEMENT_3D('',#37197,#29861,#29862);
#26472=AXIS2_PLACEMENT_3D('',#37198,#29863,#29864);
#26473=AXIS2_PLACEMENT_3D('',#37201,#29867,#29868);
#26474=AXIS2_PLACEMENT_3D('',#37202,#29869,#29870);
#26475=AXIS2_PLACEMENT_3D('',#37203,#29871,#29872);
#26476=AXIS2_PLACEMENT_3D('',#37204,#29873,#29874);
#26477=AXIS2_PLACEMENT_3D('',#37207,#29877,#29878);
#26478=AXIS2_PLACEMENT_3D('',#37208,#29879,#29880);
#26479=AXIS2_PLACEMENT_3D('',#37209,#29881,#29882);
#26480=AXIS2_PLACEMENT_3D('',#37212,#29885,#29886);
#26481=AXIS2_PLACEMENT_3D('',#37213,#29887,#29888);
#26482=AXIS2_PLACEMENT_3D('',#37216,#29891,#29892);
#26483=AXIS2_PLACEMENT_3D('',#37217,#29893,#29894);
#26484=AXIS2_PLACEMENT_3D('',#37218,#29895,#29896);
#26485=AXIS2_PLACEMENT_3D('',#37224,#29900,#29901);
#26486=AXIS2_PLACEMENT_3D('',#37225,#29902,#29903);
#26487=AXIS2_PLACEMENT_3D('',#37227,#29905,#29906);
#26488=AXIS2_PLACEMENT_3D('',#37233,#29909,#29910);
#26489=AXIS2_PLACEMENT_3D('',#37237,#29912,#29913);
#26490=AXIS2_PLACEMENT_3D('',#37241,#29915,#29916);
#26491=AXIS2_PLACEMENT_3D('',#37245,#29918,#29919);
#26492=AXIS2_PLACEMENT_3D('',#37247,#29920,#29921);
#26493=AXIS2_PLACEMENT_3D('',#37249,#29922,#29923);
#26494=AXIS2_PLACEMENT_3D('',#37253,#29925,#29926);
#26495=AXIS2_PLACEMENT_3D('',#37257,#29928,#29929);
#26496=AXIS2_PLACEMENT_3D('',#37261,#29931,#29932);
#26497=AXIS2_PLACEMENT_3D('',#37263,#29933,#29934);
#26498=AXIS2_PLACEMENT_3D('',#37265,#29935,#29936);
#26499=AXIS2_PLACEMENT_3D('',#37273,#29940,#29941);
#26500=AXIS2_PLACEMENT_3D('',#37275,#29942,#29943);
#26501=AXIS2_PLACEMENT_3D('',#37277,#29944,#29945);
#26502=AXIS2_PLACEMENT_3D('',#37281,#29947,#29948);
#26503=AXIS2_PLACEMENT_3D('',#37285,#29950,#29951);
#26504=AXIS2_PLACEMENT_3D('',#37289,#29953,#29954);
#26505=AXIS2_PLACEMENT_3D('',#37291,#29955,#29956);
#26506=AXIS2_PLACEMENT_3D('',#37293,#29957,#29958);
#26507=AXIS2_PLACEMENT_3D('',#37297,#29960,#29961);
#26508=AXIS2_PLACEMENT_3D('',#37301,#29963,#29964);
#26509=AXIS2_PLACEMENT_3D('',#37305,#29966,#29967);
#26510=AXIS2_PLACEMENT_3D('',#37312,#29972,#29973);
#26511=AXIS2_PLACEMENT_3D('',#37319,#29977,#29978);
#26512=AXIS2_PLACEMENT_3D('',#37323,#29980,#29981);
#26513=AXIS2_PLACEMENT_3D('',#37327,#29983,#29984);
#26514=AXIS2_PLACEMENT_3D('',#37331,#29986,#29987);
#26515=AXIS2_PLACEMENT_3D('',#37333,#29988,#29989);
#26516=AXIS2_PLACEMENT_3D('',#37335,#29990,#29991);
#26517=AXIS2_PLACEMENT_3D('',#37339,#29993,#29994);
#26518=AXIS2_PLACEMENT_3D('',#37343,#29996,#29997);
#26519=AXIS2_PLACEMENT_3D('',#37347,#29999,#30000);
#26520=AXIS2_PLACEMENT_3D('',#37349,#30001,#30002);
#26521=AXIS2_PLACEMENT_3D('',#37351,#30003,#30004);
#26522=AXIS2_PLACEMENT_3D('',#37359,#30008,#30009);
#26523=AXIS2_PLACEMENT_3D('',#37361,#30010,#30011);
#26524=AXIS2_PLACEMENT_3D('',#37363,#30012,#30013);
#26525=AXIS2_PLACEMENT_3D('',#37367,#30015,#30016);
#26526=AXIS2_PLACEMENT_3D('',#37371,#30018,#30019);
#26527=AXIS2_PLACEMENT_3D('',#37375,#30021,#30022);
#26528=AXIS2_PLACEMENT_3D('',#37377,#30023,#30024);
#26529=AXIS2_PLACEMENT_3D('',#37379,#30025,#30026);
#26530=AXIS2_PLACEMENT_3D('',#37383,#30028,#30029);
#26531=AXIS2_PLACEMENT_3D('',#37387,#30031,#30032);
#26532=AXIS2_PLACEMENT_3D('',#37391,#30034,#30035);
#26533=AXIS2_PLACEMENT_3D('',#37395,#30038,#30039);
#26534=AXIS2_PLACEMENT_3D('',#37398,#30042,#30043);
#26535=AXIS2_PLACEMENT_3D('',#37401,#30046,#30047);
#26536=AXIS2_PLACEMENT_3D('',#37404,#30050,#30051);
#26537=AXIS2_PLACEMENT_3D('',#37407,#30054,#30055);
#26538=AXIS2_PLACEMENT_3D('',#37410,#30058,#30059);
#26539=AXIS2_PLACEMENT_3D('',#37413,#30062,#30063);
#26540=AXIS2_PLACEMENT_3D('',#37415,#30065,#30066);
#26541=AXIS2_PLACEMENT_3D('',#37417,#30068,#30069);
#26542=AXIS2_PLACEMENT_3D('',#37419,#30071,#30072);
#26543=AXIS2_PLACEMENT_3D('',#37422,#30075,#30076);
#26544=AXIS2_PLACEMENT_3D('',#37425,#30079,#30080);
#26545=AXIS2_PLACEMENT_3D('',#37428,#30083,#30084);
#26546=AXIS2_PLACEMENT_3D('',#37431,#30087,#30088);
#26547=AXIS2_PLACEMENT_3D('',#37433,#30090,#30091);
#26548=AXIS2_PLACEMENT_3D('',#37436,#30094,#30095);
#26549=AXIS2_PLACEMENT_3D('',#37439,#30098,#30099);
#26550=AXIS2_PLACEMENT_3D('',#37440,#30100,#30101);
#26551=AXIS2_PLACEMENT_3D('',#37441,#30102,#30103);
#26552=AXIS2_PLACEMENT_3D('',#37442,#30104,#30105);
#26553=AXIS2_PLACEMENT_3D('',#37443,#30106,#30107);
#26554=AXIS2_PLACEMENT_3D('',#37444,#30108,#30109);
#26555=AXIS2_PLACEMENT_3D('',#37445,#30110,#30111);
#26556=AXIS2_PLACEMENT_3D('',#37446,#30112,#30113);
#26557=AXIS2_PLACEMENT_3D('',#37447,#30114,#30115);
#26558=AXIS2_PLACEMENT_3D('',#37448,#30116,#30117);
#26559=AXIS2_PLACEMENT_3D('',#37451,#30120,#30121);
#26560=AXIS2_PLACEMENT_3D('',#37454,#30124,#30125);
#26561=AXIS2_PLACEMENT_3D('',#37457,#30128,#30129);
#26562=AXIS2_PLACEMENT_3D('',#37460,#30132,#30133);
#26563=AXIS2_PLACEMENT_3D('',#37461,#30134,#30135);
#26564=AXIS2_PLACEMENT_3D('',#37464,#30138,#30139);
#26565=AXIS2_PLACEMENT_3D('',#37467,#30142,#30143);
#26566=AXIS2_PLACEMENT_3D('',#37468,#30144,#30145);
#26567=AXIS2_PLACEMENT_3D('',#37469,#30146,#30147);
#26568=AXIS2_PLACEMENT_3D('',#37470,#30148,#30149);
#26569=AXIS2_PLACEMENT_3D('',#37471,#30150,#30151);
#26570=AXIS2_PLACEMENT_3D('',#37472,#30152,#30153);
#26571=AXIS2_PLACEMENT_3D('',#37473,#30154,#30155);
#26572=AXIS2_PLACEMENT_3D('',#37474,#30156,#30157);
#26573=AXIS2_PLACEMENT_3D('',#37475,#30158,#30159);
#26574=AXIS2_PLACEMENT_3D('',#37476,#30160,#30161);
#26575=AXIS2_PLACEMENT_3D('',#37477,#30162,#30163);
#26576=AXIS2_PLACEMENT_3D('',#37479,#30165,#30166);
#26577=AXIS2_PLACEMENT_3D('',#37480,#30167,#30168);
#26578=AXIS2_PLACEMENT_3D('',#37481,#30169,#30170);
#26579=AXIS2_PLACEMENT_3D('',#37482,#30171,#30172);
#26580=AXIS2_PLACEMENT_3D('',#37483,#30173,#30174);
#26581=AXIS2_PLACEMENT_3D('',#37484,#30175,#30176);
#26582=AXIS2_PLACEMENT_3D('',#37485,#30177,#30178);
#26583=AXIS2_PLACEMENT_3D('',#37486,#30179,#30180);
#26584=AXIS2_PLACEMENT_3D('',#37487,#30181,#30182);
#26585=AXIS2_PLACEMENT_3D('',#37488,#30183,#30184);
#26586=AXIS2_PLACEMENT_3D('',#37489,#30185,#30186);
#26587=AXIS2_PLACEMENT_3D('',#37490,#30187,#30188);
#26588=AXIS2_PLACEMENT_3D('',#37491,#30189,#30190);
#26589=AXIS2_PLACEMENT_3D('',#37492,#30191,#30192);
#26590=AXIS2_PLACEMENT_3D('',#37493,#30193,#30194);
#26591=AXIS2_PLACEMENT_3D('',#37494,#30195,#30196);
#29287=DIRECTION('axis',(0.,0.,1.));
#29288=DIRECTION('refdir',(1.,0.,0.));
#29289=DIRECTION('center_axis',(0.,1.,0.));
#29290=DIRECTION('ref_axis',(0.,0.,1.));
#29291=DIRECTION('center_axis',(0.,1.,0.));
#29292=DIRECTION('ref_axis',(0.,0.,1.));
#29293=DIRECTION('',(0.,1.,0.));
#29294=DIRECTION('center_axis',(0.,1.,0.));
#29295=DIRECTION('ref_axis',(0.,0.,1.));
#29296=DIRECTION('center_axis',(0.,1.,0.));
#29297=DIRECTION('ref_axis',(0.,0.,1.));
#29298=DIRECTION('center_axis',(6.19544098563146E-17,1.,0.));
#29299=DIRECTION('ref_axis',(-1.,6.19544098563146E-17,0.));
#29300=DIRECTION('center_axis',(-0.707106781186749,0.707106781186346,6.63628373648637E-13));
#29301=DIRECTION('ref_axis',(0.707106781186346,0.707106781186749,2.23245825814312E-8));
#29302=DIRECTION('center_axis',(0.,1.,0.));
#29303=DIRECTION('ref_axis',(0.,0.,1.));
#29304=DIRECTION('center_axis',(-0.707106781186739,0.707106781186356,-6.35085217767548E-13));
#29305=DIRECTION('ref_axis',(0.707106781186356,0.707106781186739,4.00793704510469E-8));
#29306=DIRECTION('center_axis',(6.19544098563146E-17,1.,0.));
#29307=DIRECTION('ref_axis',(-1.,6.19544098563146E-17,0.));
#29308=DIRECTION('',(0.,1.,0.));
#29309=DIRECTION('center_axis',(0.,1.,0.));
#29310=DIRECTION('ref_axis',(0.,0.,1.));
#29311=DIRECTION('center_axis',(6.19544098563146E-17,1.,0.));
#29312=DIRECTION('ref_axis',(-1.,6.19544098563146E-17,0.));
#29313=DIRECTION('center_axis',(0.707106781186538,0.707106781186557,3.68682429798511E-14));
#29314=DIRECTION('ref_axis',(0.707106781186557,-0.707106781186538,1.32375375864267E-10));
#29315=DIRECTION('center_axis',(0.,1.,0.));
#29316=DIRECTION('ref_axis',(0.,0.,1.));
#29317=DIRECTION('center_axis',(0.707106781186323,0.707106781186772,-7.32607666957653E-13));
#29318=DIRECTION('ref_axis',(0.707106781186772,-0.707106781186323,-6.06018510665849E-9));
#29319=DIRECTION('center_axis',(0.,1.,0.));
#29320=DIRECTION('ref_axis',(0.,0.,1.));
#29321=DIRECTION('center_axis',(0.,1.,0.));
#29322=DIRECTION('ref_axis',(0.,0.,1.));
#29323=DIRECTION('',(0.,1.,0.));
#29324=DIRECTION('center_axis',(0.,1.,0.));
#29325=DIRECTION('ref_axis',(0.,0.,1.));
#29326=DIRECTION('center_axis',(0.,1.,0.));
#29327=DIRECTION('ref_axis',(0.,0.,1.));
#29328=DIRECTION('center_axis',(6.19544098563146E-17,1.,0.));
#29329=DIRECTION('ref_axis',(-1.,6.19544098563146E-17,0.));
#29330=DIRECTION('center_axis',(-0.707106781186744,0.707106781186351,6.50546093878307E-13));
#29331=DIRECTION('ref_axis',(0.707106781186351,0.707106781186744,7.42984904174717E-10));
#29332=DIRECTION('center_axis',(0.,1.,0.));
#29333=DIRECTION('ref_axis',(0.,0.,1.));
#29334=DIRECTION('center_axis',(-0.707106781186742,0.707106781186353,-6.42221006739863E-13));
#29335=DIRECTION('ref_axis',(0.707106781186353,0.707106781186742,2.97716291710107E-8));
#29336=DIRECTION('center_axis',(6.19544098563146E-17,1.,0.));
#29337=DIRECTION('ref_axis',(-1.,6.19544098563146E-17,0.));
#29338=DIRECTION('',(0.,1.,0.));
#29339=DIRECTION('center_axis',(0.,1.,0.));
#29340=DIRECTION('ref_axis',(0.,0.,1.));
#29341=DIRECTION('center_axis',(6.19544098563146E-17,1.,0.));
#29342=DIRECTION('ref_axis',(-1.,6.19544098563146E-17,0.));
#29343=DIRECTION('center_axis',(0.707106781186537,0.707106781186558,3.56789448193693E-14));
#29344=DIRECTION('ref_axis',(0.707106781186557,-0.707106781186537,-9.53308819765748E-9));
#29345=DIRECTION('center_axis',(0.,1.,0.));
#29346=DIRECTION('ref_axis',(0.,0.,1.));
#29347=DIRECTION('center_axis',(0.707106781186315,0.70710678118678,-7.56393630180537E-13));
#29348=DIRECTION('ref_axis',(0.70710678118678,-0.707106781186315,-2.44027645301359E-8));
#29349=DIRECTION('center_axis',(0.,1.,0.));
#29350=DIRECTION('ref_axis',(0.,0.,1.));
#29351=DIRECTION('center_axis',(0.,1.,0.));
#29352=DIRECTION('ref_axis',(0.,0.,1.));
#29353=DIRECTION('',(0.,1.,0.));
#29354=DIRECTION('center_axis',(0.,1.,0.));
#29355=DIRECTION('ref_axis',(0.,0.,1.));
#29356=DIRECTION('center_axis',(0.,1.,0.));
#29357=DIRECTION('ref_axis',(0.,0.,1.));
#29358=DIRECTION('center_axis',(6.19544098563146E-17,1.,0.));
#29359=DIRECTION('ref_axis',(-1.,6.19544098563146E-17,0.));
#29360=DIRECTION('center_axis',(-0.707106781186747,0.707106781186348,6.58871181003077E-13));
#29361=DIRECTION('ref_axis',(0.707106781186348,0.707106781186747,1.69840014417738E-8));
#29362=DIRECTION('center_axis',(0.,1.,0.));
#29363=DIRECTION('ref_axis',(0.,0.,1.));
#29364=DIRECTION('center_axis',(-0.707106781186741,0.707106781186354,-6.42221006748515E-13));
#29365=DIRECTION('ref_axis',(0.707106781186354,0.707106781186741,1.98080202652188E-8));
#29366=DIRECTION('center_axis',(6.19544098563146E-17,1.,0.));
#29367=DIRECTION('ref_axis',(-1.,6.19544098563146E-17,0.));
#29368=DIRECTION('',(0.,1.,0.));
#29369=DIRECTION('center_axis',(0.,1.,0.));
#29370=DIRECTION('ref_axis',(0.,0.,1.));
#29371=DIRECTION('center_axis',(6.19544098563146E-17,1.,0.));
#29372=DIRECTION('ref_axis',(-1.,6.19544098563146E-17,0.));
#29373=DIRECTION('center_axis',(0.707106781186533,0.707106781186562,4.51933301047554E-14));
#29374=DIRECTION('ref_axis',(0.707106781186562,-0.707106781186533,-3.30550302651237E-9));
#29375=DIRECTION('center_axis',(0.,1.,0.));
#29376=DIRECTION('ref_axis',(0.,0.,1.));
#29377=DIRECTION('center_axis',(0.707106781186314,0.707106781186781,-7.5639363017397E-13));
#29378=DIRECTION('ref_axis',(0.707106781186781,-0.707106781186314,-1.22471854963268E-8));
#29379=DIRECTION('center_axis',(0.,1.,0.));
#29380=DIRECTION('ref_axis',(0.,0.,1.));
#29381=DIRECTION('center_axis',(0.,1.,0.));
#29382=DIRECTION('ref_axis',(0.,0.,1.));
#29383=DIRECTION('',(0.,1.,0.));
#29384=DIRECTION('center_axis',(0.,1.,0.));
#29385=DIRECTION('ref_axis',(0.,0.,1.));
#29386=DIRECTION('center_axis',(0.,1.,0.));
#29387=DIRECTION('ref_axis',(0.,0.,1.));
#29388=DIRECTION('center_axis',(6.19544098563146E-17,1.,0.));
#29389=DIRECTION('ref_axis',(-1.,6.19544098563146E-17,0.));
#29390=DIRECTION('center_axis',(-0.707106781186749,0.707106781186347,6.60060479163914E-13));
#29391=DIRECTION('ref_axis',(0.707106781186346,0.707106781186748,2.47609223171707E-8));
#29392=DIRECTION('center_axis',(0.,1.,0.));
#29393=DIRECTION('ref_axis',(0.,0.,1.));
#29394=DIRECTION('center_axis',(-0.707106781186743,0.707106781186353,-6.44599603075256E-13));
#29395=DIRECTION('ref_axis',(0.707106781186353,0.707106781186743,7.64517967052409E-9));
#29396=DIRECTION('center_axis',(6.19544098563146E-17,1.,0.));
#29397=DIRECTION('ref_axis',(-1.,6.19544098563146E-17,0.));
#29398=DIRECTION('',(0.,1.,0.));
#29399=DIRECTION('center_axis',(0.,1.,0.));
#29400=DIRECTION('ref_axis',(0.,0.,1.));
#29401=DIRECTION('center_axis',(6.19544098563146E-17,1.,0.));
#29402=DIRECTION('ref_axis',(-1.,6.19544098563146E-17,0.));
#29403=DIRECTION('center_axis',(0.707106781186532,0.707106781186563,5.11398209079768E-14));
#29404=DIRECTION('ref_axis',(0.707106781186563,-0.707106781186532,-3.95517993196584E-9));
#29405=DIRECTION('center_axis',(0.,1.,0.));
#29406=DIRECTION('ref_axis',(0.,0.,1.));
#29407=DIRECTION('center_axis',(0.707106781186319,0.707106781186776,-7.42122052246304E-13));
#29408=DIRECTION('ref_axis',(0.707106781186776,-0.707106781186319,-4.45259227831794E-9));
#29409=DIRECTION('center_axis',(0.,1.,0.));
#29410=DIRECTION('ref_axis',(0.,0.,1.));
#29411=DIRECTION('center_axis',(0.,1.,0.));
#29412=DIRECTION('ref_axis',(0.,0.,1.));
#29413=DIRECTION('',(0.,1.,0.));
#29414=DIRECTION('center_axis',(0.,1.,0.));
#29415=DIRECTION('ref_axis',(0.,0.,1.));
#29416=DIRECTION('center_axis',(0.,1.,0.));
#29417=DIRECTION('ref_axis',(0.,0.,1.));
#29418=DIRECTION('center_axis',(6.19544098563146E-17,1.,0.));
#29419=DIRECTION('ref_axis',(-1.,6.19544098563146E-17,0.));
#29420=DIRECTION('center_axis',(-0.707106781186743,0.707106781186353,6.43410304908884E-13));
#29421=DIRECTION('ref_axis',(0.707106781186353,0.707106781186743,-5.80498325499735E-9));
#29422=DIRECTION('center_axis',(0.,1.,0.));
#29423=DIRECTION('ref_axis',(0.,0.,1.));
#29424=DIRECTION('center_axis',(-0.707106781186738,0.707106781186357,-6.32706621460411E-13));
#29425=DIRECTION('ref_axis',(0.707106781186357,0.707106781186739,7.95059306801949E-9));
#29426=DIRECTION('center_axis',(6.19544098563146E-17,1.,0.));
#29427=DIRECTION('ref_axis',(-1.,6.19544098563146E-17,0.));
#29428=DIRECTION('',(0.,1.,0.));
#29429=DIRECTION('center_axis',(0.,1.,0.));
#29430=DIRECTION('ref_axis',(0.,0.,1.));
#29431=DIRECTION('center_axis',(6.19544098563146E-17,1.,0.));
#29432=DIRECTION('ref_axis',(-1.,6.19544098563146E-17,0.));
#29433=DIRECTION('center_axis',(0.70710678118653,0.707106781186565,5.70863117107439E-14));
#29434=DIRECTION('ref_axis',(0.707106781186565,-0.70710678118653,-9.09071113315049E-9));
#29435=DIRECTION('center_axis',(0.,1.,0.));
#29436=DIRECTION('ref_axis',(0.,0.,1.));
#29437=DIRECTION('center_axis',(0.707106781186317,0.707106781186778,-7.46879244888732E-13));
#29438=DIRECTION('ref_axis',(0.707106781186778,-0.707106781186317,-1.00256530335873E-9));
#29439=DIRECTION('center_axis',(0.,1.,0.));
#29440=DIRECTION('ref_axis',(0.,0.,1.));
#29441=DIRECTION('center_axis',(0.,1.,0.));
#29442=DIRECTION('ref_axis',(0.,0.,1.));
#29443=DIRECTION('',(0.,1.,0.));
#29444=DIRECTION('center_axis',(0.,1.,0.));
#29445=DIRECTION('ref_axis',(0.,0.,1.));
#29446=DIRECTION('center_axis',(0.,1.,0.));
#29447=DIRECTION('ref_axis',(0.,0.,1.));
#29448=DIRECTION('center_axis',(6.19544098563146E-17,1.,0.));
#29449=DIRECTION('ref_axis',(-1.,6.19544098563146E-17,0.));
#29450=DIRECTION('center_axis',(-0.707106781186744,0.707106781186351,6.48167497551415E-13));
#29451=DIRECTION('ref_axis',(0.707106781186351,0.707106781186744,-6.09200717301252E-9));
#29452=DIRECTION('center_axis',(0.,1.,0.));
#29453=DIRECTION('ref_axis',(0.,0.,1.));
#29454=DIRECTION('center_axis',(-0.707106781186739,0.707106781186356,-6.35085217784288E-13));
#29455=DIRECTION('ref_axis',(0.707106781186356,0.707106781186739,2.19719109990964E-8));
#29456=DIRECTION('center_axis',(6.19544098563146E-17,1.,0.));
#29457=DIRECTION('ref_axis',(-1.,6.19544098563146E-17,0.));
#29458=DIRECTION('',(0.,1.,0.));
#29459=DIRECTION('center_axis',(0.,1.,0.));
#29460=DIRECTION('ref_axis',(0.,0.,1.));
#29461=DIRECTION('center_axis',(6.19544098563146E-17,1.,0.));
#29462=DIRECTION('ref_axis',(-1.,6.19544098563146E-17,0.));
#29463=DIRECTION('center_axis',(0.707106781186531,0.707106781186564,5.35184172289345E-14));
#29464=DIRECTION('ref_axis',(0.707106781186564,-0.707106781186531,-2.37666658604641E-9));
#29465=DIRECTION('center_axis',(0.,1.,0.));
#29466=DIRECTION('ref_axis',(0.,0.,1.));
#29467=DIRECTION('center_axis',(0.707106781186313,0.707106781186782,-7.61150822819952E-13));
#29468=DIRECTION('ref_axis',(0.707106781186782,-0.707106781186313,-1.44200498676106E-8));
#29469=DIRECTION('center_axis',(0.,1.,0.));
#29470=DIRECTION('ref_axis',(0.,0.,1.));
#29471=DIRECTION('center_axis',(0.,1.,0.));
#29472=DIRECTION('ref_axis',(0.,0.,1.));
#29473=DIRECTION('',(0.,1.,0.));
#29474=DIRECTION('center_axis',(0.,1.,0.));
#29475=DIRECTION('ref_axis',(0.,0.,1.));
#29476=DIRECTION('center_axis',(0.,1.,0.));
#29477=DIRECTION('ref_axis',(0.,0.,1.));
#29478=DIRECTION('center_axis',(6.19544098563146E-17,1.,0.));
#29479=DIRECTION('ref_axis',(-1.,6.19544098563146E-17,0.));
#29480=DIRECTION('center_axis',(-0.707106781186525,0.70710678118657,-6.42221006747096E-14));
#29481=DIRECTION('ref_axis',(0.70710678118657,0.707106781186525,-6.27115230759585E-9));
#29482=DIRECTION('center_axis',(0.,1.,0.));
#29483=DIRECTION('ref_axis',(0.,0.,1.));
#29484=DIRECTION('center_axis',(-0.707106781186519,0.707106781186576,7.84936786023992E-14));
#29485=DIRECTION('ref_axis',(0.707106781186576,0.707106781186519,-6.37187636878396E-9));
#29486=DIRECTION('center_axis',(6.19544098563146E-17,1.,0.));
#29487=DIRECTION('ref_axis',(-1.,6.19544098563146E-17,0.));
#29488=DIRECTION('',(0.,1.,0.));
#29489=DIRECTION('center_axis',(0.,1.,0.));
#29490=DIRECTION('ref_axis',(0.,0.,1.));
#29491=DIRECTION('center_axis',(6.19544098563146E-17,1.,0.));
#29492=DIRECTION('ref_axis',(-1.,6.19544098563146E-17,0.));
#29493=DIRECTION('center_axis',(0.707106781186529,0.707106781186566,5.82756098715003E-14));
#29494=DIRECTION('ref_axis',(0.707106781186566,-0.707106781186529,-1.41665956895109E-8));
#29495=DIRECTION('center_axis',(0.,1.,0.));
#29496=DIRECTION('ref_axis',(0.,0.,1.));
#29497=DIRECTION('center_axis',(0.707106781186545,0.707106781186551,-1.18929816065332E-14));
#29498=DIRECTION('ref_axis',(0.707106781186551,-0.707106781186544,8.15266177051329E-10));
#29499=DIRECTION('center_axis',(0.,1.,0.));
#29500=DIRECTION('ref_axis',(0.,0.,1.));
#29501=DIRECTION('center_axis',(0.,1.,0.));
#29502=DIRECTION('ref_axis',(0.,0.,1.));
#29503=DIRECTION('',(0.,1.,0.));
#29504=DIRECTION('center_axis',(0.,1.,0.));
#29505=DIRECTION('ref_axis',(0.,0.,1.));
#29506=DIRECTION('center_axis',(0.,1.,0.));
#29507=DIRECTION('ref_axis',(0.,0.,1.));
#29508=DIRECTION('center_axis',(6.19544098563146E-17,1.,0.));
#29509=DIRECTION('ref_axis',(-1.,6.19544098563146E-17,0.));
#29510=DIRECTION('center_axis',(-0.70710678118652,0.707106781186575,-7.61150822814556E-14));
#29511=DIRECTION('ref_axis',(0.707106781186575,0.70710678118652,-4.07577956776154E-9));
#29512=DIRECTION('center_axis',(0.,1.,0.));
#29513=DIRECTION('ref_axis',(0.,0.,1.));
#29514=DIRECTION('center_axis',(-0.707106781186515,0.70710678118658,9.0386660208839E-14));
#29515=DIRECTION('ref_axis',(0.70710678118658,0.707106781186515,-1.02669175321909E-8));
#29516=DIRECTION('center_axis',(6.19544098563146E-17,1.,0.));
#29517=DIRECTION('ref_axis',(-1.,6.19544098563146E-17,0.));
#29518=DIRECTION('',(0.,1.,0.));
#29519=DIRECTION('center_axis',(0.,1.,0.));
#29520=DIRECTION('ref_axis',(0.,0.,1.));
#29521=DIRECTION('center_axis',(6.19544098563146E-17,1.,0.));
#29522=DIRECTION('ref_axis',(-1.,6.19544098563146E-17,0.));
#29523=DIRECTION('center_axis',(0.707106781186539,0.707106781186556,2.8543155855425E-14));
#29524=DIRECTION('ref_axis',(0.707106781186556,-0.707106781186539,-4.86876680138915E-9));
#29525=DIRECTION('center_axis',(0.,1.,0.));
#29526=DIRECTION('ref_axis',(0.,0.,1.));
#29527=DIRECTION('center_axis',(0.707106781186531,0.707106781186564,-5.23291190687391E-14));
#29528=DIRECTION('ref_axis',(0.707106781186564,-0.707106781186531,-1.99327366961659E-9));
#29529=DIRECTION('center_axis',(0.,1.,0.));
#29530=DIRECTION('ref_axis',(0.,0.,1.));
#29531=DIRECTION('center_axis',(0.,1.,0.));
#29532=DIRECTION('ref_axis',(0.,0.,1.));
#29533=DIRECTION('',(0.,1.,0.));
#29534=DIRECTION('center_axis',(0.,1.,0.));
#29535=DIRECTION('ref_axis',(0.,0.,1.));
#29536=DIRECTION('center_axis',(0.,1.,0.));
#29537=DIRECTION('ref_axis',(0.,0.,1.));
#29538=DIRECTION('center_axis',(6.19544098563146E-17,1.,0.));
#29539=DIRECTION('ref_axis',(-1.,6.19544098563146E-17,0.));
#29540=DIRECTION('center_axis',(-0.707106781186522,0.707106781186573,-7.13578896385657E-14));
#29541=DIRECTION('ref_axis',(0.707106781186573,0.707106781186522,6.06499231681277E-9));
#29542=DIRECTION('center_axis',(0.,1.,0.));
#29543=DIRECTION('ref_axis',(0.,0.,1.));
#29544=DIRECTION('center_axis',(-0.707106781186519,0.707106781186576,8.08722749240661E-14));
#29545=DIRECTION('ref_axis',(0.707106781186576,0.707106781186519,-1.40864771617222E-10));
#29546=DIRECTION('center_axis',(6.19544098563146E-17,1.,0.));
#29547=DIRECTION('ref_axis',(-1.,6.19544098563146E-17,0.));
#29548=DIRECTION('',(0.,1.,0.));
#29549=DIRECTION('center_axis',(0.,1.,0.));
#29550=DIRECTION('ref_axis',(0.,0.,1.));
#29551=DIRECTION('center_axis',(6.19544098563146E-17,1.,0.));
#29552=DIRECTION('ref_axis',(-1.,6.19544098563146E-17,0.));
#29553=DIRECTION('center_axis',(0.707106781186539,0.707106781186557,3.21110503373454E-14));
#29554=DIRECTION('ref_axis',(0.707106781186556,-0.707106781186539,-4.86391357561765E-9));
#29555=DIRECTION('center_axis',(0.,1.,0.));
#29556=DIRECTION('ref_axis',(0.,0.,1.));
#29557=DIRECTION('center_axis',(0.707106781186532,0.707106781186563,-4.99505227472087E-14));
#29558=DIRECTION('ref_axis',(0.707106781186563,-0.707106781186532,-5.10750268434258E-9));
#29559=DIRECTION('center_axis',(0.,1.,0.));
#29560=DIRECTION('ref_axis',(0.,0.,1.));
#29561=DIRECTION('center_axis',(0.,1.,0.));
#29562=DIRECTION('ref_axis',(0.,0.,1.));
#29563=DIRECTION('',(0.,1.,0.));
#29564=DIRECTION('center_axis',(0.,1.,0.));
#29565=DIRECTION('ref_axis',(0.,0.,1.));
#29566=DIRECTION('center_axis',(0.,1.,0.));
#29567=DIRECTION('ref_axis',(0.,0.,1.));
#29568=DIRECTION('center_axis',(6.19544098563146E-17,1.,0.));
#29569=DIRECTION('ref_axis',(-1.,6.19544098563146E-17,0.));
#29570=DIRECTION('center_axis',(-0.707106781186522,0.707106781186573,-7.13578896387188E-14));
#29571=DIRECTION('ref_axis',(0.707106781186573,0.707106781186522,7.5295440732973E-10));
#29572=DIRECTION('center_axis',(0.,1.,0.));
#29573=DIRECTION('ref_axis',(0.,0.,1.));
#29574=DIRECTION('center_axis',(-0.707106781186517,0.707106781186578,8.32508712456219E-14));
#29575=DIRECTION('ref_axis',(0.707106781186578,0.707106781186517,-1.68444693514637E-9));
#29576=DIRECTION('center_axis',(6.19544098563146E-17,1.,0.));
#29577=DIRECTION('ref_axis',(-1.,6.19544098563146E-17,0.));
#29578=DIRECTION('',(0.,1.,0.));
#29579=DIRECTION('center_axis',(0.,1.,0.));
#29580=DIRECTION('ref_axis',(0.,0.,1.));
#29581=DIRECTION('center_axis',(6.19544098563146E-17,1.,0.));
#29582=DIRECTION('ref_axis',(-1.,6.19544098563146E-17,0.));
#29583=DIRECTION('center_axis',(0.707106781186545,0.707106781186551,1.54608760883638E-14));
#29584=DIRECTION('ref_axis',(0.70710678118655,-0.707106781186544,-3.54497137075718E-9));
#29585=DIRECTION('center_axis',(0.,1.,0.));
#29586=DIRECTION('ref_axis',(0.,0.,1.));
#29587=DIRECTION('center_axis',(0.707106781186539,0.707106781186556,-3.09217521768553E-14));
#29588=DIRECTION('ref_axis',(0.707106781186556,-0.707106781186539,-6.02871288395333E-10));
#29589=DIRECTION('center_axis',(0.,1.,0.));
#29590=DIRECTION('ref_axis',(0.,0.,1.));
#29591=DIRECTION('center_axis',(0.,1.,0.));
#29592=DIRECTION('ref_axis',(0.,0.,1.));
#29593=DIRECTION('',(0.,1.,0.));
#29594=DIRECTION('center_axis',(0.,1.,0.));
#29595=DIRECTION('ref_axis',(0.,0.,1.));
#29596=DIRECTION('center_axis',(0.,1.,0.));
#29597=DIRECTION('ref_axis',(0.,0.,1.));
#29598=DIRECTION('center_axis',(6.19544098563146E-17,1.,0.));
#29599=DIRECTION('ref_axis',(-1.,6.19544098563146E-17,0.));
#29600=DIRECTION('center_axis',(-0.707106781186537,0.707106781186558,-2.14073668916551E-14));
#29601=DIRECTION('ref_axis',(0.707106781186558,0.707106781186537,-4.91138244991823E-9));
#29602=DIRECTION('center_axis',(0.,1.,0.));
#29603=DIRECTION('ref_axis',(0.,0.,1.));
#29604=DIRECTION('center_axis',(-0.707106781186534,0.707106781186561,3.09217521768376E-14));
#29605=DIRECTION('ref_axis',(0.707106781186561,0.707106781186534,-5.32748781420606E-10));
#29606=DIRECTION('center_axis',(6.19544098563146E-17,1.,0.));
#29607=DIRECTION('ref_axis',(-1.,6.19544098563146E-17,0.));
#29608=DIRECTION('',(0.,1.,0.));
#29609=DIRECTION('center_axis',(0.,1.,0.));
#29610=DIRECTION('ref_axis',(0.,0.,1.));
#29611=DIRECTION('center_axis',(6.19544098563146E-17,1.,0.));
#29612=DIRECTION('ref_axis',(-1.,6.19544098563146E-17,0.));
#29613=DIRECTION('center_axis',(0.707106781186538,0.707106781186557,3.33003484980685E-14));
#29614=DIRECTION('ref_axis',(0.707106781186557,-0.707106781186538,-2.51785900200259E-9));
#29615=DIRECTION('center_axis',(0.,1.,0.));
#29616=DIRECTION('ref_axis',(0.,0.,1.));
#29617=DIRECTION('center_axis',(0.707106781186537,0.707106781186558,-3.56789448195543E-14));
#29618=DIRECTION('ref_axis',(0.707106781186558,-0.707106781186537,-1.21671693251198E-9));
#29619=DIRECTION('center_axis',(0.,1.,0.));
#29620=DIRECTION('ref_axis',(0.,0.,1.));
#29621=DIRECTION('center_axis',(0.,1.,0.));
#29622=DIRECTION('ref_axis',(0.,0.,1.));
#29623=DIRECTION('',(0.,1.,0.));
#29624=DIRECTION('center_axis',(0.,1.,0.));
#29625=DIRECTION('ref_axis',(0.,0.,1.));
#29626=DIRECTION('center_axis',(0.,1.,0.));
#29627=DIRECTION('ref_axis',(0.,0.,1.));
#29628=DIRECTION('center_axis',(6.19544098563146E-17,1.,0.));
#29629=DIRECTION('ref_axis',(-1.,6.19544098563146E-17,0.));
#29630=DIRECTION('center_axis',(-0.707106781186544,0.707106781186551,-1.18929816064752E-15));
#29631=DIRECTION('ref_axis',(0.707106781186551,0.707106781186544,-2.79028008532548E-9));
#29632=DIRECTION('center_axis',(0.,1.,0.));
#29633=DIRECTION('ref_axis',(0.,0.,1.));
#29634=DIRECTION('center_axis',(-0.707106781186539,0.707106781186556,1.42715779277559E-14));
#29635=DIRECTION('ref_axis',(0.707106781186556,0.707106781186539,-3.56410008544113E-9));
#29636=DIRECTION('center_axis',(6.19544098563146E-17,1.,0.));
#29637=DIRECTION('ref_axis',(-1.,6.19544098563146E-17,0.));
#29638=DIRECTION('',(0.,1.,0.));
#29639=DIRECTION('center_axis',(0.,1.,0.));
#29640=DIRECTION('ref_axis',(0.,0.,1.));
#29641=DIRECTION('center_axis',(6.19544098563146E-17,1.,0.));
#29642=DIRECTION('ref_axis',(-1.,6.19544098563146E-17,0.));
#29643=DIRECTION('center_axis',(0.707106781186545,0.707106781186551,1.42715779278094E-14));
#29644=DIRECTION('ref_axis',(0.70710678118655,-0.707106781186544,2.08661794038888E-9));
#29645=DIRECTION('center_axis',(0.,1.,0.));
#29646=DIRECTION('ref_axis',(0.,0.,1.));
#29647=DIRECTION('center_axis',(0.707106781186539,0.707106781186556,-3.09217521767969E-14));
#29648=DIRECTION('ref_axis',(0.707106781186556,-0.707106781186539,-1.0692782140686E-9));
#29649=DIRECTION('center_axis',(0.,1.,0.));
#29650=DIRECTION('ref_axis',(0.,0.,1.));
#29651=DIRECTION('center_axis',(0.,1.,0.));
#29652=DIRECTION('ref_axis',(0.,0.,1.));
#29653=DIRECTION('',(0.,1.,0.));
#29654=DIRECTION('center_axis',(0.,1.,0.));
#29655=DIRECTION('ref_axis',(0.,0.,1.));
#29656=DIRECTION('center_axis',(0.,1.,0.));
#29657=DIRECTION('ref_axis',(0.,0.,1.));
#29658=DIRECTION('center_axis',(6.19544098563146E-17,1.,0.));
#29659=DIRECTION('ref_axis',(-1.,6.19544098563146E-17,0.));
#29660=DIRECTION('center_axis',(-0.707106781186536,0.707106781186559,-2.37859632129691E-14));
#29661=DIRECTION('ref_axis',(0.707106781186559,0.707106781186536,1.5906322003989E-9));
#29662=DIRECTION('center_axis',(0.,1.,0.));
#29663=DIRECTION('ref_axis',(0.,0.,1.));
#29664=DIRECTION('center_axis',(-0.707106781186543,0.707106781186552,4.75719264259406E-15));
#29665=DIRECTION('ref_axis',(0.707106781186552,0.707106781186543,-1.87099840895288E-9));
#29666=DIRECTION('center_axis',(6.19544098563146E-17,1.,0.));
#29667=DIRECTION('ref_axis',(-1.,6.19544098563146E-17,0.));
#29668=DIRECTION('',(0.,1.,0.));
#29669=DIRECTION('center_axis',(0.,1.,0.));
#29670=DIRECTION('ref_axis',(0.,0.,1.));
#29671=DIRECTION('center_axis',(6.19544098563146E-17,1.,0.));
#29672=DIRECTION('ref_axis',(-1.,6.19544098563146E-17,0.));
#29673=DIRECTION('center_axis',(0.707106781186536,0.707106781186559,3.80575411406882E-14));
#29674=DIRECTION('ref_axis',(0.707106781186559,-0.707106781186536,-4.18851469439042E-10));
#29675=DIRECTION('center_axis',(0.,1.,0.));
#29676=DIRECTION('ref_axis',(0.,0.,1.));
#29677=DIRECTION('center_axis',(0.707106781186532,0.707106781186563,-4.99505227472632E-14));
#29678=DIRECTION('ref_axis',(0.707106781186563,-0.707106781186532,3.80158663483794E-10));
#29679=DIRECTION('center_axis',(0.,1.,0.));
#29680=DIRECTION('ref_axis',(0.,0.,1.));
#29681=DIRECTION('center_axis',(0.,1.,0.));
#29682=DIRECTION('ref_axis',(0.,0.,1.));
#29683=DIRECTION('',(0.,1.,0.));
#29684=DIRECTION('center_axis',(0.,1.,0.));
#29685=DIRECTION('ref_axis',(0.,0.,1.));
#29686=DIRECTION('center_axis',(0.,1.,0.));
#29687=DIRECTION('ref_axis',(0.,0.,1.));
#29688=DIRECTION('center_axis',(6.19544098563146E-17,1.,0.));
#29689=DIRECTION('ref_axis',(-1.,6.19544098563146E-17,0.));
#29690=DIRECTION('center_axis',(-0.707106781186545,0.707106781186551,2.37859632129592E-15));
#29691=DIRECTION('ref_axis',(0.70710678118655,0.707106781186545,4.53820074720942E-10));
#29692=DIRECTION('center_axis',(0.,1.,0.));
#29693=DIRECTION('ref_axis',(0.,0.,1.));
#29694=DIRECTION('center_axis',(-0.707106781186518,0.707106781186577,8.32508712452785E-14));
#29695=DIRECTION('ref_axis',(0.707106781186577,0.707106781186518,-3.07005203925342E-10));
#29696=DIRECTION('center_axis',(6.19544098563146E-17,1.,0.));
#29697=DIRECTION('ref_axis',(-1.,6.19544098563146E-17,0.));
#29698=DIRECTION('',(0.,1.,0.));
#29699=DIRECTION('center_axis',(0.,1.,0.));
#29700=DIRECTION('ref_axis',(0.,0.,1.));
#29701=DIRECTION('center_axis',(6.19544098563146E-17,1.,0.));
#29702=DIRECTION('ref_axis',(-1.,6.19544098563146E-17,0.));
#29703=DIRECTION('center_axis',(0.707106781186542,0.707106781186553,2.14073668916295E-14));
#29704=DIRECTION('ref_axis',(0.707106781186554,-0.707106781186542,8.8715406950362E-11));
#29705=DIRECTION('center_axis',(0.,1.,0.));
#29706=DIRECTION('ref_axis',(0.,0.,1.));
#29707=DIRECTION('center_axis',(0.707106781186542,0.707106781186553,-2.14073668916982E-14));
#29708=DIRECTION('ref_axis',(0.707106781186553,-0.707106781186542,5.58949393343591E-11));
#29709=DIRECTION('center_axis',(0.,1.,0.));
#29710=DIRECTION('ref_axis',(0.,0.,1.));
#29711=DIRECTION('center_axis',(0.,1.,0.));
#29712=DIRECTION('ref_axis',(0.,0.,1.));
#29713=DIRECTION('',(0.,1.,0.));
#29714=DIRECTION('center_axis',(0.,1.,0.));
#29715=DIRECTION('ref_axis',(0.,0.,1.));
#29716=DIRECTION('center_axis',(0.,1.,0.));
#29717=DIRECTION('ref_axis',(0.,0.,1.));
#29718=DIRECTION('center_axis',(6.19544098563146E-17,1.,0.));
#29719=DIRECTION('ref_axis',(-1.,6.19544098563146E-17,0.));
#29720=DIRECTION('center_axis',(-0.707106781186529,0.707106781186566,-4.51933301046057E-14));
#29721=DIRECTION('ref_axis',(0.707106781186566,0.707106781186529,-4.56830670056408E-11));
#29722=DIRECTION('center_axis',(0.,1.,0.));
#29723=DIRECTION('ref_axis',(0.,0.,1.));
#29724=DIRECTION('center_axis',(-0.707106781186538,0.707106781186557,1.90287705703604E-14));
#29725=DIRECTION('ref_axis',(0.707106781186557,0.707106781186538,3.34877097628957E-11));
#29726=DIRECTION('center_axis',(6.19544098563146E-17,1.,0.));
#29727=DIRECTION('ref_axis',(-1.,6.19544098563146E-17,0.));
#29728=DIRECTION('',(0.,1.,0.));
#29729=DIRECTION('center_axis',(0.,1.,0.));
#29730=DIRECTION('ref_axis',(0.,0.,1.));
#29731=DIRECTION('center_axis',(6.19544098563146E-17,1.,0.));
#29732=DIRECTION('ref_axis',(-1.,6.19544098563146E-17,0.));
#29733=DIRECTION('center_axis',(0.707106781186535,0.70710678118656,4.16254356226834E-14));
#29734=DIRECTION('ref_axis',(0.70710678118656,-0.707106781186535,-8.62446084296705E-11));
#29735=DIRECTION('center_axis',(0.,1.,0.));
#29736=DIRECTION('ref_axis',(0.,0.,1.));
#29737=DIRECTION('center_axis',(0.707106781186536,0.707106781186559,-4.04361374620356E-14));
#29738=DIRECTION('ref_axis',(0.707106781186559,-0.707106781186536,7.09281942410052E-11));
#29739=DIRECTION('center_axis',(-0.707106781186544,0.707106781186551,0.));
#29740=DIRECTION('ref_axis',(-0.707106781186551,-0.707106781186544,0.));
#29741=DIRECTION('',(0.,0.,1.));
#29742=DIRECTION('',(0.,0.,1.));
#29743=DIRECTION('',(-0.707106781186551,-0.707106781186544,0.));
#29744=DIRECTION('center_axis',(0.707106781186551,0.707106781186544,0.));
#29745=DIRECTION('ref_axis',(-0.707106781186544,0.707106781186551,0.));
#29746=DIRECTION('',(0.,0.,1.));
#29747=DIRECTION('',(0.,0.,1.));
#29748=DIRECTION('center_axis',(1.22464679914735E-16,-1.,0.));
#29749=DIRECTION('ref_axis',(1.,1.22464679914735E-16,0.));
#29750=DIRECTION('',(0.,0.,1.));
#29751=DIRECTION('',(0.,0.,1.));
#29752=DIRECTION('',(0.,0.,1.));
#29753=DIRECTION('',(0.,0.,1.));
#29754=DIRECTION('',(0.,0.,1.));
#29755=DIRECTION('',(0.,0.,1.));
#29756=DIRECTION('',(0.,0.,1.));
#29757=DIRECTION('',(0.,0.,1.));
#29758=DIRECTION('',(0.,0.,1.));
#29759=DIRECTION('',(0.,0.,1.));
#29760=DIRECTION('',(0.,0.,1.));
#29761=DIRECTION('',(0.,0.,1.));
#29762=DIRECTION('',(0.,0.,1.));
#29763=DIRECTION('',(0.,0.,1.));
#29764=DIRECTION('',(0.,0.,1.));
#29765=DIRECTION('',(1.,1.22464679914735E-16,0.));
#29766=DIRECTION('',(0.,0.,1.));
#29767=DIRECTION('',(1.,1.22464679914735E-16,0.));
#29768=DIRECTION('center_axis',(6.19544098563146E-17,1.,0.));
#29769=DIRECTION('ref_axis',(-1.,6.19544098563146E-17,0.));
#29770=DIRECTION('',(0.,0.,1.));
#29771=DIRECTION('center_axis',(1.22464679914735E-16,-1.,0.));
#29772=DIRECTION('ref_axis',(1.,1.22464679914735E-16,0.));
#29773=DIRECTION('',(0.,0.,1.));
#29774=DIRECTION('',(1.,1.22464679914735E-16,0.));
#29775=DIRECTION('',(0.,0.,1.));
#29776=DIRECTION('',(1.,1.22464679914735E-16,0.));
#29777=DIRECTION('',(0.,0.,1.));
#29778=DIRECTION('',(0.,0.,1.));
#29779=DIRECTION('',(0.,0.,1.));
#29780=DIRECTION('',(0.,0.,1.));
#29781=DIRECTION('',(0.,0.,1.));
#29782=DIRECTION('',(0.,0.,1.));
#29783=DIRECTION('',(0.,0.,1.));
#29784=DIRECTION('',(0.,0.,1.));
#29785=DIRECTION('',(0.,0.,1.));
#29786=DIRECTION('',(0.,0.,1.));
#29787=DIRECTION('',(0.,0.,1.));
#29788=DIRECTION('',(0.,0.,1.));
#29789=DIRECTION('',(0.,0.,1.));
#29790=DIRECTION('',(0.,0.,1.));
#29791=DIRECTION('center_axis',(-0.707106781186544,0.707106781186551,0.));
#29792=DIRECTION('ref_axis',(-0.707106781186551,-0.707106781186544,0.));
#29793=DIRECTION('center_axis',(6.19544098563146E-17,1.,0.));
#29794=DIRECTION('ref_axis',(-1.,6.19544098563146E-17,0.));
#29795=DIRECTION('',(0.,0.,1.));
#29796=DIRECTION('',(0.,0.,1.));
#29797=DIRECTION('center_axis',(0.707106781186551,0.707106781186544,0.));
#29798=DIRECTION('ref_axis',(-0.707106781186544,0.707106781186551,0.));
#29799=DIRECTION('center_axis',(-0.707106781186544,0.707106781186551,0.));
#29800=DIRECTION('ref_axis',(-0.707106781186551,-0.707106781186544,0.));
#29801=DIRECTION('center_axis',(6.19544098563146E-17,1.,0.));
#29802=DIRECTION('ref_axis',(-1.,6.19544098563146E-17,0.));
#29803=DIRECTION('',(0.,0.,1.));
#29804=DIRECTION('',(0.,0.,1.));
#29805=DIRECTION('center_axis',(0.707106781186551,0.707106781186544,0.));
#29806=DIRECTION('ref_axis',(-0.707106781186544,0.707106781186551,0.));
#29807=DIRECTION('center_axis',(-0.707106781186544,0.707106781186551,0.));
#29808=DIRECTION('ref_axis',(-0.707106781186551,-0.707106781186544,0.));
#29809=DIRECTION('center_axis',(6.19544098563146E-17,1.,0.));
#29810=DIRECTION('ref_axis',(-1.,6.19544098563146E-17,0.));
#29811=DIRECTION('',(0.,0.,1.));
#29812=DIRECTION('',(0.,0.,1.));
#29813=DIRECTION('center_axis',(0.707106781186551,0.707106781186544,0.));
#29814=DIRECTION('ref_axis',(-0.707106781186544,0.707106781186551,0.));
#29815=DIRECTION('center_axis',(-0.707106781186544,0.707106781186551,0.));
#29816=DIRECTION('ref_axis',(-0.707106781186551,-0.707106781186544,0.));
#29817=DIRECTION('center_axis',(6.19544098563146E-17,1.,0.));
#29818=DIRECTION('ref_axis',(-1.,6.19544098563146E-17,0.));
#29819=DIRECTION('',(0.,0.,1.));
#29820=DIRECTION('',(0.,0.,1.));
#29821=DIRECTION('center_axis',(0.707106781186551,0.707106781186544,0.));
#29822=DIRECTION('ref_axis',(-0.707106781186544,0.707106781186551,0.));
#29823=DIRECTION('center_axis',(-0.707106781186544,0.707106781186551,0.));
#29824=DIRECTION('ref_axis',(-0.707106781186551,-0.707106781186544,0.));
#29825=DIRECTION('center_axis',(6.19544098563146E-17,1.,0.));
#29826=DIRECTION('ref_axis',(-1.,6.19544098563146E-17,0.));
#29827=DIRECTION('',(0.,0.,1.));
#29828=DIRECTION('',(0.,0.,1.));
#29829=DIRECTION('center_axis',(0.707106781186551,0.707106781186544,0.));
#29830=DIRECTION('ref_axis',(-0.707106781186544,0.707106781186551,0.));
#29831=DIRECTION('center_axis',(-0.707106781186544,0.707106781186551,0.));
#29832=DIRECTION('ref_axis',(-0.707106781186551,-0.707106781186544,0.));
#29833=DIRECTION('center_axis',(6.19544098563146E-17,1.,0.));
#29834=DIRECTION('ref_axis',(-1.,6.19544098563146E-17,0.));
#29835=DIRECTION('',(0.,0.,1.));
#29836=DIRECTION('',(0.,0.,1.));
#29837=DIRECTION('center_axis',(0.707106781186551,0.707106781186544,0.));
#29838=DIRECTION('ref_axis',(-0.707106781186544,0.707106781186551,0.));
#29839=DIRECTION('center_axis',(-0.707106781186544,0.707106781186551,0.));
#29840=DIRECTION('ref_axis',(-0.707106781186551,-0.707106781186544,0.));
#29841=DIRECTION('center_axis',(6.19544098563146E-17,1.,0.));
#29842=DIRECTION('ref_axis',(-1.,6.19544098563146E-17,0.));
#29843=DIRECTION('',(0.,0.,1.));
#29844=DIRECTION('',(0.,0.,1.));
#29845=DIRECTION('center_axis',(0.707106781186551,0.707106781186544,0.));
#29846=DIRECTION('ref_axis',(-0.707106781186544,0.707106781186551,0.));
#29847=DIRECTION('center_axis',(-0.707106781186544,0.707106781186551,0.));
#29848=DIRECTION('ref_axis',(-0.707106781186551,-0.707106781186544,0.));
#29849=DIRECTION('center_axis',(6.19544098563146E-17,1.,0.));
#29850=DIRECTION('ref_axis',(-1.,6.19544098563146E-17,0.));
#29851=DIRECTION('',(0.,0.,1.));
#29852=DIRECTION('',(0.,0.,1.));
#29853=DIRECTION('center_axis',(0.707106781186551,0.707106781186544,0.));
#29854=DIRECTION('ref_axis',(-0.707106781186544,0.707106781186551,0.));
#29855=DIRECTION('center_axis',(-0.707106781186544,0.707106781186551,0.));
#29856=DIRECTION('ref_axis',(-0.707106781186551,-0.707106781186544,0.));
#29857=DIRECTION('center_axis',(6.19544098563146E-17,1.,0.));
#29858=DIRECTION('ref_axis',(-1.,6.19544098563146E-17,0.));
#29859=DIRECTION('',(0.,0.,1.));
#29860=DIRECTION('',(0.,0.,1.));
#29861=DIRECTION('center_axis',(0.707106781186551,0.707106781186544,0.));
#29862=DIRECTION('ref_axis',(-0.707106781186544,0.707106781186551,0.));
#29863=DIRECTION('center_axis',(6.19544098563146E-17,1.,0.));
#29864=DIRECTION('ref_axis',(-1.,6.19544098563146E-17,0.));
#29865=DIRECTION('',(0.,0.,1.));
#29866=DIRECTION('',(0.,0.,1.));
#29867=DIRECTION('center_axis',(-0.707106781186544,0.707106781186551,0.));
#29868=DIRECTION('ref_axis',(-0.707106781186551,-0.707106781186544,0.));
#29869=DIRECTION('center_axis',(0.707106781186551,0.707106781186544,0.));
#29870=DIRECTION('ref_axis',(-0.707106781186544,0.707106781186551,0.));
#29871=DIRECTION('center_axis',(-0.707106781186544,0.707106781186551,0.));
#29872=DIRECTION('ref_axis',(-0.707106781186551,-0.707106781186544,0.));
#29873=DIRECTION('center_axis',(6.19544098563146E-17,1.,0.));
#29874=DIRECTION('ref_axis',(-1.,6.19544098563146E-17,0.));
#29875=DIRECTION('',(0.,0.,1.));
#29876=DIRECTION('',(0.,0.,1.));
#29877=DIRECTION('center_axis',(0.707106781186551,0.707106781186544,0.));
#29878=DIRECTION('ref_axis',(-0.707106781186544,0.707106781186551,0.));
#29879=DIRECTION('center_axis',(-0.707106781186544,0.707106781186551,0.));
#29880=DIRECTION('ref_axis',(-0.707106781186551,-0.707106781186544,0.));
#29881=DIRECTION('center_axis',(6.19544098563146E-17,1.,0.));
#29882=DIRECTION('ref_axis',(-1.,6.19544098563146E-17,0.));
#29883=DIRECTION('',(0.,0.,1.));
#29884=DIRECTION('',(0.,0.,1.));
#29885=DIRECTION('center_axis',(0.707106781186551,0.707106781186544,0.));
#29886=DIRECTION('ref_axis',(-0.707106781186544,0.707106781186551,0.));
#29887=DIRECTION('center_axis',(6.19544098563146E-17,1.,0.));
#29888=DIRECTION('ref_axis',(-1.,6.19544098563146E-17,0.));
#29889=DIRECTION('',(0.,0.,1.));
#29890=DIRECTION('',(0.,0.,1.));
#29891=DIRECTION('center_axis',(-0.707106781186544,0.707106781186551,0.));
#29892=DIRECTION('ref_axis',(-0.707106781186551,-0.707106781186544,0.));
#29893=DIRECTION('center_axis',(0.707106781186551,0.707106781186544,0.));
#29894=DIRECTION('ref_axis',(-0.707106781186544,0.707106781186551,0.));
#29895=DIRECTION('center_axis',(6.19544098563146E-17,1.,0.));
#29896=DIRECTION('ref_axis',(-1.,6.19544098563146E-17,0.));
#29897=DIRECTION('',(0.,0.,1.));
#29898=DIRECTION('',(0.,0.,1.));
#29899=DIRECTION('',(-1.,6.19544098563146E-17,0.));
#29900=DIRECTION('center_axis',(-0.707106781186544,0.707106781186551,0.));
#29901=DIRECTION('ref_axis',(-0.707106781186551,-0.707106781186544,0.));
#29902=DIRECTION('center_axis',(0.707106781186551,0.707106781186544,0.));
#29903=DIRECTION('ref_axis',(-0.707106781186544,0.707106781186551,0.));
#29904=DIRECTION('',(-0.707106781186544,0.707106781186551,0.));
#29905=DIRECTION('center_axis',(0.,0.,-1.));
#29906=DIRECTION('ref_axis',(-1.,0.,0.));
#29907=DIRECTION('',(0.707106781186544,-0.707106781186551,0.));
#29908=DIRECTION('',(0.,-1.,0.));
#29909=DIRECTION('center_axis',(0.,0.,-1.));
#29910=DIRECTION('ref_axis',(-1.,0.,0.));
#29911=DIRECTION('',(-0.707106781186551,-0.707106781186544,0.));
#29912=DIRECTION('center_axis',(0.,0.,1.));
#29913=DIRECTION('ref_axis',(-1.,0.,0.));
#29914=DIRECTION('',(0.,-1.,0.));
#29915=DIRECTION('center_axis',(0.,0.,1.));
#29916=DIRECTION('ref_axis',(-1.,0.,0.));
#29917=DIRECTION('',(0.707106781186544,-0.707106781186551,0.));
#29918=DIRECTION('center_axis',(0.,0.,-1.));
#29919=DIRECTION('ref_axis',(-1.,0.,0.));
#29920=DIRECTION('center_axis',(0.,0.,1.));
#29921=DIRECTION('ref_axis',(1.,0.,0.));
#29922=DIRECTION('center_axis',(0.,0.,-1.));
#29923=DIRECTION('ref_axis',(-1.,0.,0.));
#29924=DIRECTION('',(0.707106781186544,-0.707106781186551,0.));
#29925=DIRECTION('center_axis',(0.,0.,-1.));
#29926=DIRECTION('ref_axis',(-1.,0.,0.));
#29927=DIRECTION('',(0.,-1.,0.));
#29928=DIRECTION('center_axis',(0.,0.,-1.));
#29929=DIRECTION('ref_axis',(-1.,0.,0.));
#29930=DIRECTION('',(-0.70710678118655,-0.707106781186545,0.));
#29931=DIRECTION('center_axis',(0.,0.,-1.));
#29932=DIRECTION('ref_axis',(-1.,0.,0.));
#29933=DIRECTION('center_axis',(0.,0.,1.));
#29934=DIRECTION('ref_axis',(1.,0.,0.));
#29935=DIRECTION('center_axis',(0.,0.,-1.));
#29936=DIRECTION('ref_axis',(-1.,0.,0.));
#29937=DIRECTION('',(-0.70710678118655,-0.707106781186545,0.));
#29938=DIRECTION('',(-1.,0.,0.));
#29939=DIRECTION('',(0.70710678118655,-0.707106781186545,0.));
#29940=DIRECTION('center_axis',(0.,0.,-1.));
#29941=DIRECTION('ref_axis',(-1.,0.,0.));
#29942=DIRECTION('center_axis',(0.,0.,-1.));
#29943=DIRECTION('ref_axis',(-1.,0.,0.));
#29944=DIRECTION('center_axis',(0.,0.,-1.));
#29945=DIRECTION('ref_axis',(-1.,0.,0.));
#29946=DIRECTION('',(0.70710678118655,-0.707106781186545,0.));
#29947=DIRECTION('center_axis',(0.,0.,-1.));
#29948=DIRECTION('ref_axis',(-1.,0.,0.));
#29949=DIRECTION('',(0.,-1.,0.));
#29950=DIRECTION('center_axis',(0.,0.,-1.));
#29951=DIRECTION('ref_axis',(-1.,0.,0.));
#29952=DIRECTION('',(-0.707106781186544,-0.707106781186551,0.));
#29953=DIRECTION('center_axis',(0.,0.,-1.));
#29954=DIRECTION('ref_axis',(-1.,0.,0.));
#29955=DIRECTION('center_axis',(0.,0.,-1.));
#29956=DIRECTION('ref_axis',(-1.,0.,0.));
#29957=DIRECTION('center_axis',(0.,0.,-1.));
#29958=DIRECTION('ref_axis',(-1.,0.,0.));
#29959=DIRECTION('',(-0.707106781186544,-0.707106781186551,0.));
#29960=DIRECTION('center_axis',(0.,0.,1.));
#29961=DIRECTION('ref_axis',(-1.,-3.46944695195361E-15,0.));
#29962=DIRECTION('',(0.,-1.,0.));
#29963=DIRECTION('center_axis',(0.,0.,1.));
#29964=DIRECTION('ref_axis',(-1.,0.,0.));
#29965=DIRECTION('',(0.707106781186551,-0.707106781186544,0.));
#29966=DIRECTION('center_axis',(0.,0.,-1.));
#29967=DIRECTION('ref_axis',(-1.,0.,0.));
#29968=DIRECTION('',(0.,-1.,0.));
#29969=DIRECTION('',(-0.707106781186544,-0.707106781186551,0.));
#29970=DIRECTION('',(-0.707106781186544,0.707106781186551,0.));
#29971=DIRECTION('',(-1.,6.19544098563146E-17,0.));
#29972=DIRECTION('center_axis',(0.,0.,-1.));
#29973=DIRECTION('ref_axis',(-1.,0.,0.));
#29974=DIRECTION('',(-0.707106781186551,-0.707106781186544,0.));
#29975=DIRECTION('',(-0.707106781186544,-0.707106781186551,0.));
#29976=DIRECTION('',(0.,-1.,0.));
#29977=DIRECTION('center_axis',(0.,0.,1.));
#29978=DIRECTION('ref_axis',(-1.,1.73472347597681E-15,0.));
#29979=DIRECTION('',(0.707106781186551,-0.707106781186544,0.));
#29980=DIRECTION('center_axis',(0.,0.,-1.));
#29981=DIRECTION('ref_axis',(-1.,0.,0.));
#29982=DIRECTION('',(0.,-1.,0.));
#29983=DIRECTION('center_axis',(0.,0.,-1.));
#29984=DIRECTION('ref_axis',(-1.,0.,0.));
#29985=DIRECTION('',(-0.707106781186544,-0.707106781186551,0.));
#29986=DIRECTION('center_axis',(0.,0.,1.));
#29987=DIRECTION('ref_axis',(-1.,0.,0.));
#29988=DIRECTION('center_axis',(0.,0.,-1.));
#29989=DIRECTION('ref_axis',(-1.,0.,0.));
#29990=DIRECTION('center_axis',(0.,0.,1.));
#29991=DIRECTION('ref_axis',(-1.,-6.93889390390722E-15,0.));
#29992=DIRECTION('',(-0.707106781186544,-0.707106781186551,0.));
#29993=DIRECTION('center_axis',(0.,0.,1.));
#29994=DIRECTION('ref_axis',(-1.,0.,0.));
#29995=DIRECTION('',(0.,-1.,0.));
#29996=DIRECTION('center_axis',(0.,0.,1.));
#29997=DIRECTION('ref_axis',(-1.,0.,0.));
#29998=DIRECTION('',(0.70710678118655,-0.707106781186545,0.));
#29999=DIRECTION('center_axis',(0.,0.,1.));
#30000=DIRECTION('ref_axis',(-1.,0.,0.));
#30001=DIRECTION('center_axis',(0.,0.,-1.));
#30002=DIRECTION('ref_axis',(-1.,0.,0.));
#30003=DIRECTION('center_axis',(0.,0.,1.));
#30004=DIRECTION('ref_axis',(-1.,0.,0.));
#30005=DIRECTION('',(0.70710678118655,-0.707106781186545,0.));
#30006=DIRECTION('',(-1.,0.,0.));
#30007=DIRECTION('',(-0.70710678118655,-0.707106781186545,0.));
#30008=DIRECTION('center_axis',(0.,0.,1.));
#30009=DIRECTION('ref_axis',(-1.,0.,0.));
#30010=DIRECTION('center_axis',(0.,0.,1.));
#30011=DIRECTION('ref_axis',(1.,0.,0.));
#30012=DIRECTION('center_axis',(0.,0.,1.));
#30013=DIRECTION('ref_axis',(-1.,-6.93889390390722E-15,0.));
#30014=DIRECTION('',(-0.70710678118655,-0.707106781186545,0.));
#30015=DIRECTION('center_axis',(0.,0.,1.));
#30016=DIRECTION('ref_axis',(-1.,6.93889390390722E-15,0.));
#30017=DIRECTION('',(0.,-1.,0.));
#30018=DIRECTION('center_axis',(0.,0.,1.));
#30019=DIRECTION('ref_axis',(-1.,0.,0.));
#30020=DIRECTION('',(0.707106781186544,-0.707106781186551,0.));
#30021=DIRECTION('center_axis',(0.,0.,1.));
#30022=DIRECTION('ref_axis',(-1.,0.,0.));
#30023=DIRECTION('center_axis',(0.,0.,1.));
#30024=DIRECTION('ref_axis',(1.,0.,0.));
#30025=DIRECTION('center_axis',(0.,0.,1.));
#30026=DIRECTION('ref_axis',(-1.,0.,0.));
#30027=DIRECTION('',(0.707106781186544,-0.707106781186551,0.));
#30028=DIRECTION('center_axis',(0.,0.,-1.));
#30029=DIRECTION('ref_axis',(-1.,0.,0.));
#30030=DIRECTION('',(0.,-1.,0.));
#30031=DIRECTION('center_axis',(0.,0.,-1.));
#30032=DIRECTION('ref_axis',(-1.,0.,0.));
#30033=DIRECTION('',(-0.707106781186551,-0.707106781186544,0.));
#30034=DIRECTION('center_axis',(0.,0.,1.));
#30035=DIRECTION('ref_axis',(-1.,1.12757025938492E-14,0.));
#30036=DIRECTION('',(0.,-1.,0.));
#30037=DIRECTION('',(0.707106781186544,-0.707106781186551,0.));
#30038=DIRECTION('center_axis',(-0.70710678118655,0.707106781186545,0.));
#30039=DIRECTION('ref_axis',(-0.707106781186545,-0.70710678118655,0.));
#30040=DIRECTION('',(0.,0.,-1.));
#30041=DIRECTION('',(0.,0.,1.));
#30042=DIRECTION('center_axis',(-0.70710678118655,0.707106781186545,0.));
#30043=DIRECTION('ref_axis',(-0.707106781186545,-0.70710678118655,0.));
#30044=DIRECTION('',(0.,0.,1.));
#30045=DIRECTION('',(0.,0.,-1.));
#30046=DIRECTION('center_axis',(-0.707106781186545,-0.70710678118655,0.));
#30047=DIRECTION('ref_axis',(0.70710678118655,-0.707106781186545,0.));
#30048=DIRECTION('',(0.,0.,1.));
#30049=DIRECTION('',(0.,0.,-1.));
#30050=DIRECTION('center_axis',(-0.707106781186545,-0.70710678118655,0.));
#30051=DIRECTION('ref_axis',(0.70710678118655,-0.707106781186545,0.));
#30052=DIRECTION('',(0.,0.,-1.));
#30053=DIRECTION('',(0.,0.,1.));
#30054=DIRECTION('center_axis',(-0.70710678118655,-0.707106781186545,0.));
#30055=DIRECTION('ref_axis',(0.707106781186545,-0.70710678118655,0.));
#30056=DIRECTION('',(0.,0.,1.));
#30057=DIRECTION('',(0.,0.,-1.));
#30058=DIRECTION('center_axis',(-0.707106781186545,0.70710678118655,0.));
#30059=DIRECTION('ref_axis',(-0.70710678118655,-0.707106781186545,0.));
#30060=DIRECTION('',(0.,0.,-1.));
#30061=DIRECTION('',(0.,0.,1.));
#30062=DIRECTION('center_axis',(0.,1.,0.));
#30063=DIRECTION('ref_axis',(0.,0.,1.));
#30064=DIRECTION('',(0.,0.,1.));
#30065=DIRECTION('center_axis',(-0.707106781186551,-0.707106781186544,0.));
#30066=DIRECTION('ref_axis',(0.707106781186544,-0.707106781186551,0.));
#30067=DIRECTION('',(0.,0.,1.));
#30068=DIRECTION('center_axis',(-1.,0.,0.));
#30069=DIRECTION('ref_axis',(0.,0.,1.));
#30070=DIRECTION('',(0.,0.,-1.));
#30071=DIRECTION('center_axis',(-0.707106781186544,0.707106781186551,0.));
#30072=DIRECTION('ref_axis',(-0.707106781186551,-0.707106781186544,0.));
#30073=DIRECTION('',(0.,0.,1.));
#30074=DIRECTION('',(0.,0.,-1.));
#30075=DIRECTION('center_axis',(-1.,0.,0.));
#30076=DIRECTION('ref_axis',(0.,0.,1.));
#30077=DIRECTION('',(0.,0.,1.));
#30078=DIRECTION('',(0.,0.,-1.));
#30079=DIRECTION('center_axis',(-0.70710678118655,-0.707106781186545,0.));
#30080=DIRECTION('ref_axis',(0.707106781186545,-0.70710678118655,0.));
#30081=DIRECTION('',(0.,0.,-1.));
#30082=DIRECTION('',(0.,0.,1.));
#30083=DIRECTION('center_axis',(-1.,0.,0.));
#30084=DIRECTION('ref_axis',(0.,0.,1.));
#30085=DIRECTION('',(0.,0.,-1.));
#30086=DIRECTION('',(0.,0.,1.));
#30087=DIRECTION('center_axis',(-0.707106781186545,0.70710678118655,0.));
#30088=DIRECTION('ref_axis',(-0.70710678118655,-0.707106781186545,0.));
#30089=DIRECTION('',(0.,0.,1.));
#30090=DIRECTION('center_axis',(0.,0.,1.));
#30091=DIRECTION('ref_axis',(1.,0.,0.));
#30092=DIRECTION('',(0.,0.,1.));
#30093=DIRECTION('',(0.,0.,-1.));
#30094=DIRECTION('center_axis',(0.,0.,1.));
#30095=DIRECTION('ref_axis',(1.,0.,0.));
#30096=DIRECTION('',(0.,0.,-1.));
#30097=DIRECTION('',(0.,0.,1.));
#30098=DIRECTION('center_axis',(0.,0.,1.));
#30099=DIRECTION('ref_axis',(1.,0.,0.));
#30100=DIRECTION('center_axis',(0.,0.,1.));
#30101=DIRECTION('ref_axis',(1.,0.,0.));
#30102=DIRECTION('center_axis',(0.,0.,1.));
#30103=DIRECTION('ref_axis',(1.,0.,0.));
#30104=DIRECTION('center_axis',(0.,0.,1.));
#30105=DIRECTION('ref_axis',(1.,0.,0.));
#30106=DIRECTION('center_axis',(0.,0.,-1.));
#30107=DIRECTION('ref_axis',(-1.,0.,0.));
#30108=DIRECTION('center_axis',(0.,0.,-1.));
#30109=DIRECTION('ref_axis',(-1.,0.,0.));
#30110=DIRECTION('center_axis',(0.,0.,1.));
#30111=DIRECTION('ref_axis',(1.,0.,0.));
#30112=DIRECTION('center_axis',(0.,0.,1.));
#30113=DIRECTION('ref_axis',(1.,0.,0.));
#30114=DIRECTION('center_axis',(0.,0.,1.));
#30115=DIRECTION('ref_axis',(1.,0.,0.));
#30116=DIRECTION('center_axis',(-1.,0.,0.));
#30117=DIRECTION('ref_axis',(0.,0.,1.));
#30118=DIRECTION('',(0.,0.,1.));
#30119=DIRECTION('',(0.,0.,-1.));
#30120=DIRECTION('center_axis',(-1.,0.,0.));
#30121=DIRECTION('ref_axis',(0.,0.,1.));
#30122=DIRECTION('',(0.,0.,-1.));
#30123=DIRECTION('',(0.,0.,1.));
#30124=DIRECTION('center_axis',(-0.707106781186544,-0.707106781186551,0.));
#30125=DIRECTION('ref_axis',(0.707106781186551,-0.707106781186544,0.));
#30126=DIRECTION('',(0.,0.,-1.));
#30127=DIRECTION('',(0.,0.,1.));
#30128=DIRECTION('center_axis',(-1.,0.,0.));
#30129=DIRECTION('ref_axis',(0.,0.,1.));
#30130=DIRECTION('',(0.,0.,1.));
#30131=DIRECTION('',(0.,0.,1.));
#30132=DIRECTION('center_axis',(-0.707106781186551,0.707106781186544,0.));
#30133=DIRECTION('ref_axis',(-0.707106781186544,-0.707106781186551,0.));
#30134=DIRECTION('center_axis',(0.,0.,1.));
#30135=DIRECTION('ref_axis',(1.,0.,0.));
#30136=DIRECTION('',(0.,0.,-1.));
#30137=DIRECTION('',(0.,0.,1.));
#30138=DIRECTION('center_axis',(0.,0.,1.));
#30139=DIRECTION('ref_axis',(1.,0.,0.));
#30140=DIRECTION('',(0.,0.,1.));
#30141=DIRECTION('',(0.,0.,-1.));
#30142=DIRECTION('center_axis',(0.,0.,1.));
#30143=DIRECTION('ref_axis',(1.,0.,0.));
#30144=DIRECTION('center_axis',(0.,0.,1.));
#30145=DIRECTION('ref_axis',(1.,0.,0.));
#30146=DIRECTION('center_axis',(0.,0.,1.));
#30147=DIRECTION('ref_axis',(1.,0.,0.));
#30148=DIRECTION('center_axis',(0.,0.,1.));
#30149=DIRECTION('ref_axis',(1.,0.,0.));
#30150=DIRECTION('center_axis',(0.,0.,-1.));
#30151=DIRECTION('ref_axis',(-1.,0.,0.));
#30152=DIRECTION('center_axis',(0.,0.,-1.));
#30153=DIRECTION('ref_axis',(-1.,0.,0.));
#30154=DIRECTION('center_axis',(0.,0.,1.));
#30155=DIRECTION('ref_axis',(1.,0.,0.));
#30156=DIRECTION('center_axis',(0.,0.,1.));
#30157=DIRECTION('ref_axis',(1.,0.,0.));
#30158=DIRECTION('center_axis',(0.,0.,1.));
#30159=DIRECTION('ref_axis',(1.,0.,0.));
#30160=DIRECTION('center_axis',(-0.707106781186544,0.707106781186551,0.));
#30161=DIRECTION('ref_axis',(-0.707106781186551,-0.707106781186544,0.));
#30162=DIRECTION('center_axis',(6.19544098563146E-17,1.,0.));
#30163=DIRECTION('ref_axis',(-1.,6.19544098563146E-17,0.));
#30164=DIRECTION('',(0.,0.,1.));
#30165=DIRECTION('center_axis',(0.707106781186551,0.707106781186544,0.));
#30166=DIRECTION('ref_axis',(-0.707106781186544,0.707106781186551,0.));
#30167=DIRECTION('center_axis',(0.,-1.,0.));
#30168=DIRECTION('ref_axis',(0.,0.,-1.));
#30169=DIRECTION('center_axis',(0.,-1.,0.));
#30170=DIRECTION('ref_axis',(0.,0.,-1.));
#30171=DIRECTION('center_axis',(0.,-1.,0.));
#30172=DIRECTION('ref_axis',(0.,0.,-1.));
#30173=DIRECTION('center_axis',(0.,-1.,0.));
#30174=DIRECTION('ref_axis',(0.,0.,-1.));
#30175=DIRECTION('center_axis',(0.,-1.,0.));
#30176=DIRECTION('ref_axis',(0.,0.,-1.));
#30177=DIRECTION('center_axis',(0.,-1.,0.));
#30178=DIRECTION('ref_axis',(0.,0.,-1.));
#30179=DIRECTION('center_axis',(0.,-1.,0.));
#30180=DIRECTION('ref_axis',(0.,0.,-1.));
#30181=DIRECTION('center_axis',(0.,-1.,0.));
#30182=DIRECTION('ref_axis',(0.,0.,-1.));
#30183=DIRECTION('center_axis',(0.,-1.,0.));
#30184=DIRECTION('ref_axis',(0.,0.,-1.));
#30185=DIRECTION('center_axis',(0.,-1.,0.));
#30186=DIRECTION('ref_axis',(0.,0.,-1.));
#30187=DIRECTION('center_axis',(0.,-1.,0.));
#30188=DIRECTION('ref_axis',(0.,0.,-1.));
#30189=DIRECTION('center_axis',(0.,-1.,0.));
#30190=DIRECTION('ref_axis',(0.,0.,-1.));
#30191=DIRECTION('center_axis',(0.,-1.,0.));
#30192=DIRECTION('ref_axis',(0.,0.,-1.));
#30193=DIRECTION('center_axis',(0.,-1.,0.));
#30194=DIRECTION('ref_axis',(0.,0.,-1.));
#30195=DIRECTION('center_axis',(0.,-1.,0.));
#30196=DIRECTION('ref_axis',(0.,0.,-1.));
#36676=CARTESIAN_POINT('',(0.,0.,0.));
#36677=CARTESIAN_POINT('Origin',(0.,22.,-840.));
#36678=CARTESIAN_POINT('',(-6.73555739531038E-16,13.,-845.5));
#36679=CARTESIAN_POINT('Origin',(0.,13.,-840.));
#36680=CARTESIAN_POINT('',(-6.73555739531038E-16,22.,-845.5));
#36681=CARTESIAN_POINT('',(-6.73555739531038E-16,22.,-845.5));
#36682=CARTESIAN_POINT('Origin',(0.,22.,-840.));
#36683=CARTESIAN_POINT('Origin',(0.,22.,-840.));
#36684=CARTESIAN_POINT('',(-1.75,0.500000000000001,-836.968911086755));
#36685=CARTESIAN_POINT('',(1.75,0.5,-836.968911086755));
#36686=CARTESIAN_POINT('Origin',(0.,0.5,-840.));
#36687=CARTESIAN_POINT('',(-2.25000000000004,0.,-837.319048676309));
#36688=CARTESIAN_POINT('Origin',(-6.72148608993339E-8,2.24999993278898,
-839.999999903682));
#36689=CARTESIAN_POINT('',(-2.25000000000004,0.,-842.680951323691));
#36690=CARTESIAN_POINT('Origin',(0.,0.,-840.));
#36691=CARTESIAN_POINT('',(-1.75,0.500000000000001,-843.031088913246));
#36692=CARTESIAN_POINT('Origin',(1.20611344800459E-7,2.25000012061502,-839.999999826881));
#36693=CARTESIAN_POINT('',(-4.28626379701574E-16,0.499999999999998,-843.5));
#36694=CARTESIAN_POINT('Origin',(0.,0.5,-840.));
#36695=CARTESIAN_POINT('',(-4.28626379701567E-16,13.,-843.5));
#36696=CARTESIAN_POINT('',(-4.28626379701567E-16,22.,-843.5));
#36697=CARTESIAN_POINT('Origin',(0.,13.,-840.));
#36698=CARTESIAN_POINT('',(1.75,0.5,-843.031088913246));
#36699=CARTESIAN_POINT('Origin',(0.,0.5,-840.));
#36700=CARTESIAN_POINT('',(2.25,0.,-842.680951323691));
#36701=CARTESIAN_POINT('Origin',(4.35037561530294E-10,2.24999999956476,
-840.000000000521));
#36702=CARTESIAN_POINT('',(2.24999999999995,0.,-837.319048676309));
#36703=CARTESIAN_POINT('Origin',(0.,0.,-840.));
#36704=CARTESIAN_POINT('Origin',(1.82089687772446E-8,2.24999998178678,-839.999999973692));
#36705=CARTESIAN_POINT('Origin',(0.,22.,-780.));
#36706=CARTESIAN_POINT('',(-6.73555739531038E-16,13.,-785.5));
#36707=CARTESIAN_POINT('Origin',(0.,13.,-780.));
#36708=CARTESIAN_POINT('',(-6.73555739531038E-16,22.,-785.5));
#36709=CARTESIAN_POINT('',(-6.73555739531038E-16,22.,-785.5));
#36710=CARTESIAN_POINT('Origin',(0.,22.,-780.));
#36711=CARTESIAN_POINT('Origin',(0.,22.,-780.));
#36712=CARTESIAN_POINT('',(-1.75,0.500000000000001,-776.968911086755));
#36713=CARTESIAN_POINT('',(1.75,0.5,-776.968911086755));
#36714=CARTESIAN_POINT('Origin',(0.,0.5,-780.));
#36715=CARTESIAN_POINT('',(-2.25000000000004,0.,-777.319048676309));
#36716=CARTESIAN_POINT('Origin',(-2.60525212514295E-9,2.24999999739851,
-779.99999999796));
#36717=CARTESIAN_POINT('',(-2.25000000000004,0.,-782.680951323691));
#36718=CARTESIAN_POINT('Origin',(0.,0.,-780.));
#36719=CARTESIAN_POINT('',(-1.75,0.500000000000001,-783.031088913246));
#36720=CARTESIAN_POINT('Origin',(8.94748081181618E-8,2.25000008947852,-779.999999871003));
#36721=CARTESIAN_POINT('',(-4.28626379701574E-16,0.499999999999998,-783.5));
#36722=CARTESIAN_POINT('Origin',(0.,0.5,-780.));
#36723=CARTESIAN_POINT('',(-4.28626379701567E-16,13.,-783.5));
#36724=CARTESIAN_POINT('',(-4.28626379701567E-16,22.,-783.5));
#36725=CARTESIAN_POINT('Origin',(0.,13.,-780.));
#36726=CARTESIAN_POINT('',(1.75,0.5,-783.031088913246));
#36727=CARTESIAN_POINT('Origin',(0.,0.5,-780.));
#36728=CARTESIAN_POINT('',(2.25,0.,-782.680951323691));
#36729=CARTESIAN_POINT('Origin',(-2.84421083907027E-8,2.2500000284419,-779.999999958075));
#36730=CARTESIAN_POINT('',(2.24999999999995,0.,-777.319048676309));
#36731=CARTESIAN_POINT('Origin',(0.,0.,-780.));
#36732=CARTESIAN_POINT('Origin',(7.35978125665504E-8,2.24999992639779,-779.99999989504));
#36733=CARTESIAN_POINT('Origin',(0.,22.,-720.));
#36734=CARTESIAN_POINT('',(-6.73555739531038E-16,13.,-725.5));
#36735=CARTESIAN_POINT('Origin',(0.,13.,-720.));
#36736=CARTESIAN_POINT('',(-6.73555739531038E-16,22.,-725.5));
#36737=CARTESIAN_POINT('',(-6.73555739531038E-16,22.,-725.5));
#36738=CARTESIAN_POINT('Origin',(0.,22.,-720.));
#36739=CARTESIAN_POINT('Origin',(0.,22.,-720.));
#36740=CARTESIAN_POINT('',(-1.75,0.500000000000001,-716.968911086754));
#36741=CARTESIAN_POINT('',(1.75,0.5,-716.968911086754));
#36742=CARTESIAN_POINT('Origin',(0.,0.5,-720.));
#36743=CARTESIAN_POINT('',(-2.25000000000004,0.,-717.319048676309));
#36744=CARTESIAN_POINT('Origin',(-5.15937745304562E-8,2.24999994841004,
-719.999999928058));
#36745=CARTESIAN_POINT('',(-2.25000000000004,0.,-722.680951323691));
#36746=CARTESIAN_POINT('Origin',(0.,0.,-720.));
#36747=CARTESIAN_POINT('',(-1.75,0.500000000000001,-723.031088913246));
#36748=CARTESIAN_POINT('Origin',(5.95435789563226E-8,2.25000005954729,-719.999999914124));
#36749=CARTESIAN_POINT('',(-4.28626379701574E-16,0.499999999999998,-723.5));
#36750=CARTESIAN_POINT('Origin',(0.,0.5,-720.));
#36751=CARTESIAN_POINT('',(-4.28626379701567E-16,13.,-723.5));
#36752=CARTESIAN_POINT('',(-4.28626379701567E-16,22.,-723.5));
#36753=CARTESIAN_POINT('Origin',(0.,13.,-720.));
#36754=CARTESIAN_POINT('',(1.75,0.5,-723.031088913246));
#36755=CARTESIAN_POINT('Origin',(0.,0.5,-720.));
#36756=CARTESIAN_POINT('',(2.25,0.,-722.680951323691));
#36757=CARTESIAN_POINT('Origin',(-9.57767809506294E-9,2.25000000957741,
-719.9999999846));
#36758=CARTESIAN_POINT('',(2.24999999999995,0.,-717.319048676309));
#36759=CARTESIAN_POINT('Origin',(0.,0.,-720.));
#36760=CARTESIAN_POINT('Origin',(3.69489749907359E-8,2.24999996304662,-719.999999947332));
#36761=CARTESIAN_POINT('Origin',(0.,22.,-660.));
#36762=CARTESIAN_POINT('',(-6.73555739531038E-16,13.,-665.5));
#36763=CARTESIAN_POINT('Origin',(0.,13.,-660.));
#36764=CARTESIAN_POINT('',(-6.73555739531038E-16,22.,-665.5));
#36765=CARTESIAN_POINT('',(-6.73555739531038E-16,22.,-665.5));
#36766=CARTESIAN_POINT('Origin',(0.,22.,-660.));
#36767=CARTESIAN_POINT('Origin',(0.,22.,-660.));
#36768=CARTESIAN_POINT('',(-1.75,0.500000000000001,-656.968911086754));
#36769=CARTESIAN_POINT('',(1.75,0.5,-656.968911086754));
#36770=CARTESIAN_POINT('Origin',(0.,0.5,-660.));
#36771=CARTESIAN_POINT('',(-2.25000000000004,0.,-657.319048676309));
#36772=CARTESIAN_POINT('Origin',(-7.48657963400845E-8,2.24999992513803,
-659.999999894045));
#36773=CARTESIAN_POINT('',(-2.25000000000004,0.,-662.680951323691));
#36774=CARTESIAN_POINT('Origin',(0.,0.,-660.));
#36775=CARTESIAN_POINT('',(-1.75,0.500000000000001,-663.031088913246));
#36776=CARTESIAN_POINT('Origin',(2.28832450210881E-8,2.25000002288697,-659.999999966479));
#36777=CARTESIAN_POINT('',(-4.28626379701574E-16,0.499999999999998,-663.5));
#36778=CARTESIAN_POINT('Origin',(0.,0.5,-660.));
#36779=CARTESIAN_POINT('',(-4.28626379701567E-16,13.,-663.5));
#36780=CARTESIAN_POINT('',(-4.28626379701567E-16,22.,-663.5));
#36781=CARTESIAN_POINT('Origin',(0.,13.,-660.));
#36782=CARTESIAN_POINT('',(1.75,0.5,-663.031088913246));
#36783=CARTESIAN_POINT('Origin',(0.,0.5,-660.));
#36784=CARTESIAN_POINT('',(2.25,0.,-662.680951323691));
#36785=CARTESIAN_POINT('Origin',(-1.19103271689625E-8,2.25000001191003,
-659.999999982899));
#36786=CARTESIAN_POINT('',(2.24999999999995,0.,-657.319048676309));
#36787=CARTESIAN_POINT('Origin',(0.,0.,-660.));
#36788=CARTESIAN_POINT('Origin',(1.36341934964257E-8,2.24999998636149,-659.999999981457));
#36789=CARTESIAN_POINT('Origin',(0.,22.,-600.));
#36790=CARTESIAN_POINT('',(-6.73555739531038E-16,13.,-605.5));
#36791=CARTESIAN_POINT('Origin',(0.,13.,-600.));
#36792=CARTESIAN_POINT('',(-6.73555739531038E-16,22.,-605.5));
#36793=CARTESIAN_POINT('',(-6.73555739531038E-16,22.,-605.5));
#36794=CARTESIAN_POINT('Origin',(0.,22.,-600.));
#36795=CARTESIAN_POINT('Origin',(0.,22.,-600.));
#36796=CARTESIAN_POINT('',(-1.75,0.500000000000001,-596.968911086754));
#36797=CARTESIAN_POINT('',(1.75,0.5,-596.968911086754));
#36798=CARTESIAN_POINT('Origin',(0.,0.5,-600.));
#36799=CARTESIAN_POINT('',(-2.25000000000004,0.,-597.319048676309));
#36800=CARTESIAN_POINT('Origin',(1.7384990669278E-8,2.25000001738872,-600.000000025331));
#36801=CARTESIAN_POINT('',(-2.25000000000004,0.,-602.680951323691));
#36802=CARTESIAN_POINT('Origin',(0.,0.,-600.));
#36803=CARTESIAN_POINT('',(-1.75,0.500000000000001,-603.031088913246));
#36804=CARTESIAN_POINT('Origin',(2.39434153059825E-8,2.25000002394707,-599.999999965723));
#36805=CARTESIAN_POINT('',(-4.28626379701574E-16,0.499999999999998,-603.5));
#36806=CARTESIAN_POINT('Origin',(0.,0.5,-600.));
#36807=CARTESIAN_POINT('',(-4.28626379701567E-16,13.,-603.5));
#36808=CARTESIAN_POINT('',(-4.28626379701567E-16,22.,-603.5));
#36809=CARTESIAN_POINT('Origin',(0.,13.,-600.));
#36810=CARTESIAN_POINT('',(1.75,0.5,-603.031088913246));
#36811=CARTESIAN_POINT('Origin',(0.,0.5,-600.));
#36812=CARTESIAN_POINT('',(2.25,0.,-602.680951323691));
#36813=CARTESIAN_POINT('Origin',(-2.74330147487234E-8,2.25000002743268,
-599.999999960943));
#36814=CARTESIAN_POINT('',(2.24999999999995,0.,-597.319048676309));
#36815=CARTESIAN_POINT('Origin',(0.,0.,-600.));
#36816=CARTESIAN_POINT('Origin',(2.99699681738375E-9,2.24999999699866,-599.999999995609));
#36817=CARTESIAN_POINT('Origin',(0.,22.,-540.));
#36818=CARTESIAN_POINT('',(-6.73555739531038E-16,13.,-545.5));
#36819=CARTESIAN_POINT('Origin',(0.,13.,-540.));
#36820=CARTESIAN_POINT('',(-6.73555739531038E-16,22.,-545.5));
#36821=CARTESIAN_POINT('',(-6.73555739531038E-16,22.,-545.5));
#36822=CARTESIAN_POINT('Origin',(0.,22.,-540.));
#36823=CARTESIAN_POINT('Origin',(0.,22.,-540.));
#36824=CARTESIAN_POINT('',(-1.75,0.500000000000001,-536.968911086754));
#36825=CARTESIAN_POINT('',(1.75,0.5,-536.968911086754));
#36826=CARTESIAN_POINT('Origin',(0.,0.5,-540.));
#36827=CARTESIAN_POINT('',(-2.25000000000004,0.,-537.319048676309));
#36828=CARTESIAN_POINT('Origin',(1.84421247717559E-8,2.25000001844588,-540.000000026007));
#36829=CARTESIAN_POINT('',(-2.25000000000004,0.,-542.680951323691));
#36830=CARTESIAN_POINT('Origin',(0.,0.,-540.));
#36831=CARTESIAN_POINT('',(-1.75,0.500000000000001,-543.031088913246));
#36832=CARTESIAN_POINT('Origin',(6.61566706972039E-8,2.25000006616034,-539.999999905105));
#36833=CARTESIAN_POINT('',(-4.28626379701574E-16,0.499999999999998,-543.5));
#36834=CARTESIAN_POINT('Origin',(0.,0.5,-540.));
#36835=CARTESIAN_POINT('',(-4.28626379701567E-16,13.,-543.5));
#36836=CARTESIAN_POINT('',(-4.28626379701567E-16,22.,-543.5));
#36837=CARTESIAN_POINT('Origin',(0.,13.,-540.));
#36838=CARTESIAN_POINT('',(1.75,0.5,-543.031088913246));
#36839=CARTESIAN_POINT('Origin',(0.,0.5,-540.));
#36840=CARTESIAN_POINT('',(2.25,0.,-542.680951323691));
#36841=CARTESIAN_POINT('Origin',(-7.42096994965635E-9,2.25000000742066,
-539.999999990521));
#36842=CARTESIAN_POINT('',(2.24999999999995,0.,-537.319048676309));
#36843=CARTESIAN_POINT('Origin',(0.,0.,-540.));
#36844=CARTESIAN_POINT('Origin',(4.35878827476088E-8,2.24999995640769,-539.999999938266));
#36845=CARTESIAN_POINT('Origin',(0.,22.,-480.));
#36846=CARTESIAN_POINT('',(-6.73555739531045E-16,13.,-485.5));
#36847=CARTESIAN_POINT('Origin',(0.,13.,-480.));
#36848=CARTESIAN_POINT('',(-6.73555739531045E-16,22.,-485.5));
#36849=CARTESIAN_POINT('',(-6.73555739531045E-16,22.,-485.5));
#36850=CARTESIAN_POINT('Origin',(0.,22.,-480.));
#36851=CARTESIAN_POINT('Origin',(0.,22.,-480.));
#36852=CARTESIAN_POINT('',(-1.75,0.500000000000001,-476.968911086754));
#36853=CARTESIAN_POINT('',(1.75,0.5,-476.968911086754));
#36854=CARTESIAN_POINT('Origin',(0.,0.5,-480.));
#36855=CARTESIAN_POINT('',(-2.25,0.,-477.319048676309));
#36856=CARTESIAN_POINT('Origin',(1.90741897276858E-8,2.2500000190738,-480.000000026514));
#36857=CARTESIAN_POINT('',(-2.25,0.,-482.680951323691));
#36858=CARTESIAN_POINT('Origin',(0.,0.,-480.));
#36859=CARTESIAN_POINT('',(-1.75,0.500000000000001,-483.031088913246));
#36860=CARTESIAN_POINT('Origin',(-1.93385135682789E-8,2.24999998066101,
-480.000000027097));
#36861=CARTESIAN_POINT('',(-4.28626379701572E-16,0.499999999999998,-483.5));
#36862=CARTESIAN_POINT('Origin',(0.,0.5,-480.));
#36863=CARTESIAN_POINT('',(-4.28626379701574E-16,13.,-483.5));
#36864=CARTESIAN_POINT('',(-4.28626379701574E-16,22.,-483.5));
#36865=CARTESIAN_POINT('Origin',(0.,13.,-480.));
#36866=CARTESIAN_POINT('',(1.75,0.5,-483.031088913246));
#36867=CARTESIAN_POINT('Origin',(0.,0.5,-480.));
#36868=CARTESIAN_POINT('',(2.25,0.,-482.680951323691));
#36869=CARTESIAN_POINT('Origin',(-4.27040211525842E-8,2.25000004270368,
-479.99999993896));
#36870=CARTESIAN_POINT('',(2.25,0.,-477.319048676309));
#36871=CARTESIAN_POINT('Origin',(0.,0.,-480.));
#36872=CARTESIAN_POINT('Origin',(-2.40762548786577E-9,2.25000000240756,
-480.000000003701));
#36873=CARTESIAN_POINT('Origin',(0.,22.,-420.));
#36874=CARTESIAN_POINT('',(-6.73555739531045E-16,13.,-425.5));
#36875=CARTESIAN_POINT('Origin',(0.,13.,-420.));
#36876=CARTESIAN_POINT('',(-6.73555739531045E-16,22.,-425.5));
#36877=CARTESIAN_POINT('',(-6.73555739531045E-16,22.,-425.5));
#36878=CARTESIAN_POINT('Origin',(0.,22.,-420.));
#36879=CARTESIAN_POINT('Origin',(0.,22.,-420.));
#36880=CARTESIAN_POINT('',(-1.75,0.500000000000001,-416.968911086754));
#36881=CARTESIAN_POINT('',(1.75,0.5,-416.968911086754));
#36882=CARTESIAN_POINT('Origin',(0.,0.5,-420.));
#36883=CARTESIAN_POINT('',(-2.25,0.,-417.319048676309));
#36884=CARTESIAN_POINT('Origin',(1.23725557577004E-8,2.25000001237209,-420.000000017334));
#36885=CARTESIAN_POINT('',(-2.25,0.,-422.680951323691));
#36886=CARTESIAN_POINT('Origin',(0.,0.,-420.));
#36887=CARTESIAN_POINT('',(-1.75,0.500000000000001,-423.031088913246));
#36888=CARTESIAN_POINT('Origin',(-3.09946213139511E-8,2.24999996900483,
-420.000000044132));
#36889=CARTESIAN_POINT('',(-4.28626379701572E-16,0.499999999999998,-423.5));
#36890=CARTESIAN_POINT('Origin',(0.,0.5,-420.));
#36891=CARTESIAN_POINT('',(-4.28626379701574E-16,13.,-423.5));
#36892=CARTESIAN_POINT('',(-4.28626379701574E-16,22.,-423.5));
#36893=CARTESIAN_POINT('Origin',(0.,13.,-420.));
#36894=CARTESIAN_POINT('',(1.75,0.5,-423.031088913246));
#36895=CARTESIAN_POINT('Origin',(0.,0.5,-420.));
#36896=CARTESIAN_POINT('',(2.25,-2.16840434497101E-16,-422.680951323691));
#36897=CARTESIAN_POINT('Origin',(-1.4602281606102E-8,2.25000001460212,-419.999999978837));
#36898=CARTESIAN_POINT('',(2.25,-2.16840434497101E-16,-417.319048676309));
#36899=CARTESIAN_POINT('Origin',(0.,0.,-420.));
#36900=CARTESIAN_POINT('Origin',(5.91723503529096E-9,2.24999999408246,-419.999999991203));
#36901=CARTESIAN_POINT('Origin',(0.,22.,-360.));
#36902=CARTESIAN_POINT('',(-6.73555739531045E-16,13.,-365.5));
#36903=CARTESIAN_POINT('Origin',(0.,13.,-360.));
#36904=CARTESIAN_POINT('',(-6.73555739531045E-16,22.,-365.5));
#36905=CARTESIAN_POINT('',(-6.73555739531045E-16,22.,-365.5));
#36906=CARTESIAN_POINT('Origin',(0.,22.,-360.));
#36907=CARTESIAN_POINT('Origin',(0.,22.,-360.));
#36908=CARTESIAN_POINT('',(-1.75,0.500000000000001,-356.968911086754));
#36909=CARTESIAN_POINT('',(1.75,0.5,-356.968911086754));
#36910=CARTESIAN_POINT('Origin',(0.,0.5,-360.));
#36911=CARTESIAN_POINT('',(-2.25,0.,-357.319048676309));
#36912=CARTESIAN_POINT('Origin',(-1.82331699738469E-8,2.2499999817664,-359.999999973701));
#36913=CARTESIAN_POINT('',(-2.25,0.,-362.680951323691));
#36914=CARTESIAN_POINT('Origin',(0.,0.,-360.));
#36915=CARTESIAN_POINT('',(-1.75,0.500000000000001,-363.031088913246));
#36916=CARTESIAN_POINT('Origin',(-4.38715175299365E-10,2.2499999995608,
-360.000000000543));
#36917=CARTESIAN_POINT('',(-4.28626379701572E-16,0.499999999999998,-363.5));
#36918=CARTESIAN_POINT('Origin',(0.,0.5,-360.));
#36919=CARTESIAN_POINT('',(-4.28626379701574E-16,13.,-363.5));
#36920=CARTESIAN_POINT('',(-4.28626379701574E-16,22.,-363.5));
#36921=CARTESIAN_POINT('Origin',(0.,13.,-360.));
#36922=CARTESIAN_POINT('',(1.75,0.5,-363.031088913246));
#36923=CARTESIAN_POINT('Origin',(0.,0.5,-360.));
#36924=CARTESIAN_POINT('',(2.25,-2.16840434497101E-16,-362.680951323691));
#36925=CARTESIAN_POINT('Origin',(-1.45931708384062E-8,2.25000001459299,
-359.999999978876));
#36926=CARTESIAN_POINT('',(2.25,-2.16840434497101E-16,-357.319048676309));
#36927=CARTESIAN_POINT('Origin',(0.,0.,-360.));
#36928=CARTESIAN_POINT('Origin',(1.5377042417164E-8,2.24999998462267,-359.999999977933));
#36929=CARTESIAN_POINT('Origin',(0.,22.,-300.));
#36930=CARTESIAN_POINT('',(-6.73555739531045E-16,13.,-305.5));
#36931=CARTESIAN_POINT('Origin',(0.,13.,-300.));
#36932=CARTESIAN_POINT('',(-6.73555739531045E-16,22.,-305.5));
#36933=CARTESIAN_POINT('',(-6.73555739531045E-16,22.,-305.5));
#36934=CARTESIAN_POINT('Origin',(0.,22.,-300.));
#36935=CARTESIAN_POINT('Origin',(0.,22.,-300.));
#36936=CARTESIAN_POINT('',(-1.75,0.500000000000001,-296.968911086754));
#36937=CARTESIAN_POINT('',(1.75,0.5,-296.968911086754));
#36938=CARTESIAN_POINT('Origin',(0.,0.5,-300.));
#36939=CARTESIAN_POINT('',(-2.25,0.,-297.319048676309));
#36940=CARTESIAN_POINT('Origin',(-2.37414948811576E-9,2.24999999762542,
-299.999999997033));
#36941=CARTESIAN_POINT('',(-2.25,0.,-302.680951323691));
#36942=CARTESIAN_POINT('Origin',(0.,0.,-300.));
#36943=CARTESIAN_POINT('',(-1.75,0.500000000000001,-303.031088913246));
#36944=CARTESIAN_POINT('Origin',(-5.11385406243292E-9,2.24999999488564,
-300.000000007122));
#36945=CARTESIAN_POINT('',(-4.28626379701572E-16,0.499999999999998,-303.5));
#36946=CARTESIAN_POINT('Origin',(0.,0.5,-300.));
#36947=CARTESIAN_POINT('',(-4.28626379701574E-16,13.,-303.5));
#36948=CARTESIAN_POINT('',(-4.28626379701574E-16,22.,-303.5));
#36949=CARTESIAN_POINT('Origin',(0.,13.,-300.));
#36950=CARTESIAN_POINT('',(1.75,0.5,-303.031088913245));
#36951=CARTESIAN_POINT('Origin',(0.,0.5,-300.));
#36952=CARTESIAN_POINT('',(2.25,-2.16840434497101E-16,-302.680951323691));
#36953=CARTESIAN_POINT('Origin',(-1.07341244226511E-8,2.25000001073404,
-299.999999984895));
#36954=CARTESIAN_POINT('',(2.25,-2.16840434497101E-16,-297.319048676309));
#36955=CARTESIAN_POINT('Origin',(0.,0.,-300.));
#36956=CARTESIAN_POINT('Origin',(1.81055004322417E-9,2.24999999818928,-299.999999997399));
#36957=CARTESIAN_POINT('Origin',(0.,22.,-240.));
#36958=CARTESIAN_POINT('',(-6.73555739531045E-16,13.,-245.5));
#36959=CARTESIAN_POINT('Origin',(0.,13.,-240.));
#36960=CARTESIAN_POINT('',(-6.73555739531045E-16,22.,-245.5));
#36961=CARTESIAN_POINT('',(-6.73555739531045E-16,22.,-245.5));
#36962=CARTESIAN_POINT('Origin',(0.,22.,-240.));
#36963=CARTESIAN_POINT('Origin',(0.,22.,-240.));
#36964=CARTESIAN_POINT('',(-1.75,0.500000000000001,-236.968911086754));
#36965=CARTESIAN_POINT('',(1.75,0.5,-236.968911086754));
#36966=CARTESIAN_POINT('Origin',(0.,0.5,-240.));
#36967=CARTESIAN_POINT('',(-2.25,0.,-237.319048676309));
#36968=CARTESIAN_POINT('Origin',(1.47928452820523E-8,2.2500000147927,-240.000000021201));
#36969=CARTESIAN_POINT('',(-2.25,0.,-242.680951323691));
#36970=CARTESIAN_POINT('Origin',(0.,0.,-240.));
#36971=CARTESIAN_POINT('',(-1.75,0.500000000000001,-243.031088913246));
#36972=CARTESIAN_POINT('Origin',(-1.55246204780468E-9,2.24999999844734,
-240.000000002442));
#36973=CARTESIAN_POINT('',(-4.28626379701572E-16,0.499999999999998,-243.5));
#36974=CARTESIAN_POINT('Origin',(0.,0.5,-240.));
#36975=CARTESIAN_POINT('',(-4.28626379701574E-16,13.,-243.5));
#36976=CARTESIAN_POINT('',(-4.28626379701574E-16,22.,-243.5));
#36977=CARTESIAN_POINT('Origin',(0.,13.,-240.));
#36978=CARTESIAN_POINT('',(1.75,0.5,-243.031088913246));
#36979=CARTESIAN_POINT('Origin',(0.,0.5,-240.));
#36980=CARTESIAN_POINT('',(2.25,-2.16840434497101E-16,-242.680951323691));
#36981=CARTESIAN_POINT('Origin',(-7.64266927522073E-9,2.25000000764248,
-239.99999998931));
#36982=CARTESIAN_POINT('',(2.25,-2.16840434497101E-16,-237.319048676309));
#36983=CARTESIAN_POINT('Origin',(0.,0.,-240.));
#36984=CARTESIAN_POINT('Origin',(3.72062075593149E-9,2.24999999627917,-239.999999994952));
#36985=CARTESIAN_POINT('Origin',(0.,22.,-180.));
#36986=CARTESIAN_POINT('',(-6.73555739531045E-16,13.,-185.5));
#36987=CARTESIAN_POINT('Origin',(0.,13.,-180.));
#36988=CARTESIAN_POINT('',(-6.73555739531045E-16,22.,-185.5));
#36989=CARTESIAN_POINT('',(-6.73555739531045E-16,22.,-185.5));
#36990=CARTESIAN_POINT('Origin',(0.,22.,-180.));
#36991=CARTESIAN_POINT('Origin',(0.,22.,-180.));
#36992=CARTESIAN_POINT('',(-1.75,0.500000000000001,-176.968911086754));
#36993=CARTESIAN_POINT('',(1.75,0.5,-176.968911086755));
#36994=CARTESIAN_POINT('Origin',(0.,0.5,-180.));
#36995=CARTESIAN_POINT('',(-2.25000000000001,0.,-177.319048676309));
#36996=CARTESIAN_POINT('Origin',(8.34885383049766E-9,2.25000000834883,-180.000000012206));
#36997=CARTESIAN_POINT('',(-2.25000000000001,0.,-182.680951323691));
#36998=CARTESIAN_POINT('Origin',(0.,0.,-180.));
#36999=CARTESIAN_POINT('',(-1.75,0.500000000000001,-183.031088913246));
#37000=CARTESIAN_POINT('Origin',(-1.07031097873467E-8,2.24999998929679,
-180.00000001549));
#37001=CARTESIAN_POINT('',(-4.28626379701572E-16,0.499999999999998,-183.5));
#37002=CARTESIAN_POINT('Origin',(0.,0.5,-180.));
#37003=CARTESIAN_POINT('',(-4.28626379701574E-16,13.,-183.5));
#37004=CARTESIAN_POINT('',(-4.28626379701574E-16,22.,-183.5));
#37005=CARTESIAN_POINT('Origin',(0.,13.,-180.));
#37006=CARTESIAN_POINT('',(1.75,0.5,-183.031088913246));
#37007=CARTESIAN_POINT('Origin',(0.,0.5,-180.));
#37008=CARTESIAN_POINT('',(2.25,-2.16840434497101E-16,-182.680951323691));
#37009=CARTESIAN_POINT('Origin',(6.25733659331829E-9,2.24999999374259,-180.000000009063));
#37010=CARTESIAN_POINT('',(2.25,-2.16840434497101E-16,-177.319048676309));
#37011=CARTESIAN_POINT('Origin',(0.,0.,-180.));
#37012=CARTESIAN_POINT('Origin',(3.19985427044145E-9,2.24999999679997,-179.999999995321));
#37013=CARTESIAN_POINT('Origin',(0.,22.,-120.));
#37014=CARTESIAN_POINT('',(-6.73555739531045E-16,13.,-125.5));
#37015=CARTESIAN_POINT('Origin',(0.,13.,-120.));
#37016=CARTESIAN_POINT('',(-6.73555739531045E-16,22.,-125.5));
#37017=CARTESIAN_POINT('',(-6.73555739531045E-16,22.,-125.5));
#37018=CARTESIAN_POINT('Origin',(0.,22.,-120.));
#37019=CARTESIAN_POINT('Origin',(0.,22.,-120.));
#37020=CARTESIAN_POINT('',(-1.75,0.500000000000001,-116.968911086754));
#37021=CARTESIAN_POINT('',(1.75,0.5,-116.968911086754));
#37022=CARTESIAN_POINT('Origin',(0.,0.5,-120.));
#37023=CARTESIAN_POINT('',(-2.25000000000001,0.,-117.319048676309));
#37024=CARTESIAN_POINT('Origin',(-4.79071532444308E-9,2.24999999520912,
-119.999999993143));
#37025=CARTESIAN_POINT('',(-2.25000000000001,0.,-122.680951323691));
#37026=CARTESIAN_POINT('Origin',(0.,0.,-120.));
#37027=CARTESIAN_POINT('',(-1.75,0.500000000000001,-123.031088913246));
#37028=CARTESIAN_POINT('Origin',(-5.64915392242682E-9,2.2499999943508,-120.000000008031));
#37029=CARTESIAN_POINT('',(-4.28626379701574E-16,0.499999999999998,-123.5));
#37030=CARTESIAN_POINT('Origin',(0.,0.5,-120.));
#37031=CARTESIAN_POINT('',(-4.28626379701574E-16,13.,-123.5));
#37032=CARTESIAN_POINT('',(-4.28626379701574E-16,22.,-123.5));
#37033=CARTESIAN_POINT('Origin',(0.,13.,-120.));
#37034=CARTESIAN_POINT('',(1.75,0.5,-123.031088913246));
#37035=CARTESIAN_POINT('Origin',(0.,0.5,-120.));
#37036=CARTESIAN_POINT('',(2.25,-2.16840434497101E-16,-122.680951323691));
#37037=CARTESIAN_POINT('Origin',(-1.26511134901364E-9,2.25000000126489,
-119.99999999821));
#37038=CARTESIAN_POINT('',(2.25,-2.16840434497101E-16,-117.319048676309));
#37039=CARTESIAN_POINT('Origin',(0.,0.,-120.));
#37040=CARTESIAN_POINT('Origin',(-1.13244302824E-9,2.25000000113215,-120.000000001689));
#37041=CARTESIAN_POINT('Origin',(0.,22.,-60.));
#37042=CARTESIAN_POINT('',(-6.73555739531044E-16,13.,-65.5));
#37043=CARTESIAN_POINT('Origin',(0.,13.,-60.));
#37044=CARTESIAN_POINT('',(-6.73555739531044E-16,22.,-65.5));
#37045=CARTESIAN_POINT('',(-6.73555739531044E-16,22.,-65.5));
#37046=CARTESIAN_POINT('Origin',(0.,22.,-60.));
#37047=CARTESIAN_POINT('Origin',(0.,22.,-60.));
#37048=CARTESIAN_POINT('',(-1.75,0.500000000000001,-56.9689110867545));
#37049=CARTESIAN_POINT('',(1.75,0.5,-56.9689110867544));
#37050=CARTESIAN_POINT('Origin',(0.,0.5,-60.));
#37051=CARTESIAN_POINT('',(-2.25000000000001,0.,-57.3190486763091));
#37052=CARTESIAN_POINT('Origin',(-1.35908062581791E-9,2.24999999864092,
-59.9999999980204));
#37053=CARTESIAN_POINT('',(-2.25,0.,-62.6809513236909));
#37054=CARTESIAN_POINT('Origin',(0.,0.,-60.));
#37055=CARTESIAN_POINT('',(-1.75,0.500000000000001,-63.0310889132455));
#37056=CARTESIAN_POINT('Origin',(-9.11769826306141E-10,2.24999999908773,
-60.0000000013664));
#37057=CARTESIAN_POINT('',(-4.28626379701573E-16,0.499999999999998,-63.5));
#37058=CARTESIAN_POINT('Origin',(0.,0.5,-60.));
#37059=CARTESIAN_POINT('',(-4.28626379701573E-16,13.,-63.5));
#37060=CARTESIAN_POINT('',(-4.28626379701573E-16,22.,-63.5));
#37061=CARTESIAN_POINT('Origin',(0.,13.,-60.));
#37062=CARTESIAN_POINT('',(1.75,0.5,-63.0310889132455));
#37063=CARTESIAN_POINT('Origin',(0.,0.5,-60.));
#37064=CARTESIAN_POINT('',(2.25,-2.16840434497101E-16,-62.6809513236909));
#37065=CARTESIAN_POINT('Origin',(2.79500866895432E-10,2.24999999972038,
-60.0000000003599));
#37066=CARTESIAN_POINT('',(2.25,-2.16840434497101E-16,-57.3190486763091));
#37067=CARTESIAN_POINT('Origin',(0.,0.,-60.));
#37068=CARTESIAN_POINT('Origin',(-1.95772009714545E-10,2.25000000019565,
-60.0000000001797));
#37069=CARTESIAN_POINT('Origin',(0.,22.,0.));
#37070=CARTESIAN_POINT('',(-6.73555739531044E-16,13.,-5.5));
#37071=CARTESIAN_POINT('Origin',(0.,13.,0.));
#37072=CARTESIAN_POINT('',(-6.73555739531044E-16,22.,-5.5));
#37073=CARTESIAN_POINT('',(-6.73555739531044E-16,22.,-5.5));
#37074=CARTESIAN_POINT('Origin',(0.,22.,0.));
#37075=CARTESIAN_POINT('Origin',(0.,22.,0.));
#37076=CARTESIAN_POINT('',(-1.75,0.500000000000001,3.03108891324553));
#37077=CARTESIAN_POINT('',(1.75,0.5,3.03108891324555));
#37078=CARTESIAN_POINT('Origin',(0.,0.5,0.));
#37079=CARTESIAN_POINT('',(-2.25,0.,2.68095132369089));
#37080=CARTESIAN_POINT('Origin',(1.37767852681492E-10,2.25000000013748,
-1.96202498692344E-10));
#37081=CARTESIAN_POINT('',(-2.25,0.,-2.68095132369089));
#37082=CARTESIAN_POINT('Origin',(0.,0.,0.));
#37083=CARTESIAN_POINT('',(-1.75,0.500000000000001,-3.03108891324553));
#37084=CARTESIAN_POINT('Origin',(1.01115227302273E-10,2.25000000010099,
1.42931222413267E-10));
#37085=CARTESIAN_POINT('',(-4.28626379701573E-16,0.499999999999998,-3.5));
#37086=CARTESIAN_POINT('Origin',(0.,0.5,0.));
#37087=CARTESIAN_POINT('',(-4.28626379701573E-16,13.,-3.5));
#37088=CARTESIAN_POINT('',(-4.28626379701573E-16,22.,-3.5));
#37089=CARTESIAN_POINT('Origin',(0.,13.,0.));
#37090=CARTESIAN_POINT('',(1.75,0.5,-3.03108891324555));
#37091=CARTESIAN_POINT('Origin',(0.,0.5,0.));
#37092=CARTESIAN_POINT('',(2.25,-2.16840434497101E-16,-2.6809513236909));
#37093=CARTESIAN_POINT('Origin',(-2.64255839432792E-10,2.25000000026401,
3.62936902753574E-10));
#37094=CARTESIAN_POINT('',(2.25,-2.16840434497101E-16,2.6809513236909));
#37095=CARTESIAN_POINT('Origin',(0.,0.,0.));
#37096=CARTESIAN_POINT('Origin',(-2.17712237127188E-10,2.25000000021748,
-2.98289171141164E-10));
#37097=CARTESIAN_POINT('Origin',(-2.25,-1.4389599889981E-16,-870.));
#37098=CARTESIAN_POINT('',(-1.75,0.5,-870.));
#37099=CARTESIAN_POINT('',(-1.75,0.5,-870.));
#37100=CARTESIAN_POINT('',(-2.25,-1.4389599889981E-16,-870.));
#37101=CARTESIAN_POINT('',(-2.25,-1.4389599889981E-16,-870.));
#37102=CARTESIAN_POINT('',(-2.25,-1.4389599889981E-16,-870.));
#37103=CARTESIAN_POINT('Origin',(1.75,0.5,-870.));
#37104=CARTESIAN_POINT('',(1.75,0.5,-870.));
#37105=CARTESIAN_POINT('',(2.25,-1.30104260698261E-15,-870.));
#37106=CARTESIAN_POINT('Origin',(0.,0.,-870.));
#37107=CARTESIAN_POINT('',(-2.25,-1.4389599889981E-16,-870.));
#37108=CARTESIAN_POINT('',(-2.25,-1.4389599889981E-16,-870.));
#37109=CARTESIAN_POINT('',(-2.25,-1.4389599889981E-16,-870.));
#37110=CARTESIAN_POINT('',(-2.25,-1.4389599889981E-16,-870.));
#37111=CARTESIAN_POINT('',(-2.25,-1.4389599889981E-16,-870.));
#37112=CARTESIAN_POINT('',(-2.25,-1.4389599889981E-16,-870.));
#37113=CARTESIAN_POINT('',(-2.25,-1.4389599889981E-16,-870.));
#37114=CARTESIAN_POINT('',(-2.25,-1.4389599889981E-16,-870.));
#37115=CARTESIAN_POINT('',(-2.25,-1.4389599889981E-16,-870.));
#37116=CARTESIAN_POINT('',(-2.25,-1.4389599889981E-16,-870.));
#37117=CARTESIAN_POINT('',(-2.25,-1.4389599889981E-16,-870.));
#37118=CARTESIAN_POINT('',(-2.25,-1.4389599889981E-16,-870.));
#37119=CARTESIAN_POINT('',(-2.25,-1.4389599889981E-16,-870.));
#37120=CARTESIAN_POINT('',(-2.25,-1.4389599889981E-16,-870.));
#37121=CARTESIAN_POINT('',(-2.25,-1.4389599889981E-16,30.));
#37122=CARTESIAN_POINT('',(-2.25,-1.4389599889981E-16,-870.));
#37123=CARTESIAN_POINT('',(-10.5,-1.28587913910472E-15,30.));
#37124=CARTESIAN_POINT('',(0.,0.,30.));
#37125=CARTESIAN_POINT('',(-10.5,-1.28587913910472E-15,-870.));
#37126=CARTESIAN_POINT('',(-10.5,-1.28587913910472E-15,-870.));
#37127=CARTESIAN_POINT('',(0.,0.,-870.));
#37128=CARTESIAN_POINT('Origin',(-1.75,0.5,-870.));
#37129=CARTESIAN_POINT('',(-1.75,0.5,-870.));
#37130=CARTESIAN_POINT('Origin',(0.,0.,-870.));
#37131=CARTESIAN_POINT('',(2.24999999999999,2.75545529808154E-16,-870.));
#37132=CARTESIAN_POINT('',(2.25,-1.30104260698261E-15,-870.));
#37133=CARTESIAN_POINT('',(10.5,-1.28587913910472E-15,-870.));
#37134=CARTESIAN_POINT('',(0.,0.,-870.));
#37135=CARTESIAN_POINT('',(10.5,-1.28587913910472E-15,30.));
#37136=CARTESIAN_POINT('',(10.5,-1.28587913910472E-15,-870.));
#37137=CARTESIAN_POINT('',(2.25,-1.30104260698261E-15,30.));
#37138=CARTESIAN_POINT('',(0.,0.,30.));
#37139=CARTESIAN_POINT('',(2.25,-1.30104260698261E-15,-870.));
#37140=CARTESIAN_POINT('',(2.25,-1.30104260698261E-15,-870.));
#37141=CARTESIAN_POINT('',(2.25,-1.30104260698261E-15,-870.));
#37142=CARTESIAN_POINT('',(2.25,-1.30104260698261E-15,-870.));
#37143=CARTESIAN_POINT('',(2.25,-1.30104260698261E-15,-870.));
#37144=CARTESIAN_POINT('',(2.25,-1.30104260698261E-15,-870.));
#37145=CARTESIAN_POINT('',(2.25,-1.30104260698261E-15,-870.));
#37146=CARTESIAN_POINT('',(2.25,-1.30104260698261E-15,-870.));
#37147=CARTESIAN_POINT('',(2.25,-1.30104260698261E-15,-870.));
#37148=CARTESIAN_POINT('',(2.25,-1.30104260698261E-15,-870.));
#37149=CARTESIAN_POINT('',(2.25,-1.30104260698261E-15,-870.));
#37150=CARTESIAN_POINT('',(2.25,-1.30104260698261E-15,-870.));
#37151=CARTESIAN_POINT('',(2.25,-1.30104260698261E-15,-870.));
#37152=CARTESIAN_POINT('',(2.25,-1.30104260698261E-15,-870.));
#37153=CARTESIAN_POINT('Origin',(-2.25,-1.4389599889981E-16,-870.));
#37154=CARTESIAN_POINT('Origin',(-1.75,0.5,-870.));
#37155=CARTESIAN_POINT('',(-1.75,0.5,-870.));
#37156=CARTESIAN_POINT('',(1.75,0.5,-870.));
#37157=CARTESIAN_POINT('Origin',(1.75,0.5,-870.));
#37158=CARTESIAN_POINT('Origin',(-2.25,-1.4389599889981E-16,-870.));
#37159=CARTESIAN_POINT('Origin',(-1.75,0.5,-870.));
#37160=CARTESIAN_POINT('',(-1.75,0.5,-870.));
#37161=CARTESIAN_POINT('',(1.75,0.5,-870.));
#37162=CARTESIAN_POINT('Origin',(1.75,0.5,-870.));
#37163=CARTESIAN_POINT('Origin',(-2.25,-1.4389599889981E-16,-870.));
#37164=CARTESIAN_POINT('Origin',(-1.75,0.5,-870.));
#37165=CARTESIAN_POINT('',(-1.75,0.5,-870.));
#37166=CARTESIAN_POINT('',(1.75,0.5,-870.));
#37167=CARTESIAN_POINT('Origin',(1.75,0.5,-870.));
#37168=CARTESIAN_POINT('Origin',(-2.25,-1.4389599889981E-16,-870.));
#37169=CARTESIAN_POINT('Origin',(-1.75,0.5,-870.));
#37170=CARTESIAN_POINT('',(-1.75,0.5,-870.));
#37171=CARTESIAN_POINT('',(1.75,0.5,-870.));
#37172=CARTESIAN_POINT('Origin',(1.75,0.5,-870.));
#37173=CARTESIAN_POINT('Origin',(-2.25,-1.4389599889981E-16,-870.));
#37174=CARTESIAN_POINT('Origin',(-1.75,0.5,-870.));
#37175=CARTESIAN_POINT('',(-1.75,0.5,-870.));
#37176=CARTESIAN_POINT('',(1.75,0.5,-870.));
#37177=CARTESIAN_POINT('Origin',(1.75,0.5,-870.));
#37178=CARTESIAN_POINT('Origin',(-2.25,-1.4389599889981E-16,-870.));
#37179=CARTESIAN_POINT('Origin',(-1.75,0.5,-870.));
#37180=CARTESIAN_POINT('',(-1.75,0.5,-870.));
#37181=CARTESIAN_POINT('',(1.75,0.5,-870.));
#37182=CARTESIAN_POINT('Origin',(1.75,0.5,-870.));
#37183=CARTESIAN_POINT('Origin',(-2.25,-1.4389599889981E-16,-870.));
#37184=CARTESIAN_POINT('Origin',(-1.75,0.5,-870.));
#37185=CARTESIAN_POINT('',(-1.75,0.5,-870.));
#37186=CARTESIAN_POINT('',(1.75,0.5,-870.));
#37187=CARTESIAN_POINT('Origin',(1.75,0.5,-870.));
#37188=CARTESIAN_POINT('Origin',(-2.25,-1.4389599889981E-16,-870.));
#37189=CARTESIAN_POINT('Origin',(-1.75,0.5,-870.));
#37190=CARTESIAN_POINT('',(-1.75,0.5,-870.));
#37191=CARTESIAN_POINT('',(1.75,0.5,-870.));
#37192=CARTESIAN_POINT('Origin',(1.75,0.5,-870.));
#37193=CARTESIAN_POINT('Origin',(-2.25,-1.4389599889981E-16,-870.));
#37194=CARTESIAN_POINT('Origin',(-1.75,0.5,-870.));
#37195=CARTESIAN_POINT('',(-1.75,0.5,-870.));
#37196=CARTESIAN_POINT('',(1.75,0.5,-870.));
#37197=CARTESIAN_POINT('Origin',(1.75,0.5,-870.));
#37198=CARTESIAN_POINT('Origin',(-1.75,0.5,-870.));
#37199=CARTESIAN_POINT('',(-1.75,0.5,-870.));
#37200=CARTESIAN_POINT('',(1.75,0.5,-870.));
#37201=CARTESIAN_POINT('Origin',(-2.25,-1.4389599889981E-16,-870.));
#37202=CARTESIAN_POINT('Origin',(1.75,0.5,-870.));
#37203=CARTESIAN_POINT('Origin',(-2.25,-1.4389599889981E-16,-870.));
#37204=CARTESIAN_POINT('Origin',(-1.75,0.5,-870.));
#37205=CARTESIAN_POINT('',(-1.75,0.5,-870.));
#37206=CARTESIAN_POINT('',(1.75,0.5,-870.));
#37207=CARTESIAN_POINT('Origin',(1.75,0.5,-870.));
#37208=CARTESIAN_POINT('Origin',(-2.25,-1.4389599889981E-16,-870.));
#37209=CARTESIAN_POINT('Origin',(-1.75,0.5,-870.));
#37210=CARTESIAN_POINT('',(-1.75,0.5,-870.));
#37211=CARTESIAN_POINT('',(1.75,0.5,-870.));
#37212=CARTESIAN_POINT('Origin',(1.75,0.5,-870.));
#37213=CARTESIAN_POINT('Origin',(-1.75,0.5,-870.));
#37214=CARTESIAN_POINT('',(-1.75,0.5,-870.));
#37215=CARTESIAN_POINT('',(1.75,0.5,-870.));
#37216=CARTESIAN_POINT('Origin',(-2.25,-1.4389599889981E-16,-870.));
#37217=CARTESIAN_POINT('Origin',(1.75,0.5,-870.));
#37218=CARTESIAN_POINT('Origin',(-1.75,0.5,-870.));
#37219=CARTESIAN_POINT('',(-1.75,0.5,30.));
#37220=CARTESIAN_POINT('',(-1.75,0.5,-870.));
#37221=CARTESIAN_POINT('',(1.75,0.5,30.));
#37222=CARTESIAN_POINT('',(1.75,0.5,-870.));
#37223=CARTESIAN_POINT('',(-1.75,0.5,30.));
#37224=CARTESIAN_POINT('Origin',(-2.25,-1.4389599889981E-16,-870.));
#37225=CARTESIAN_POINT('Origin',(1.75,0.5,-870.));
#37226=CARTESIAN_POINT('',(1.75,0.5,30.));
#37227=CARTESIAN_POINT('Origin',(0.,0.,-870.));
#37228=CARTESIAN_POINT('',(-11.5,1.00000000000001,-870.));
#37229=CARTESIAN_POINT('',(-10.5,-1.28587913910472E-15,-870.));
#37230=CARTESIAN_POINT('',(-11.5,5.8257864376269,-870.));
#37231=CARTESIAN_POINT('',(-11.5,1.00000000000001,-870.));
#37232=CARTESIAN_POINT('',(-11.2071067811865,6.53289321881345,-870.));
#37233=CARTESIAN_POINT('Origin',(-10.5,5.8257864376269,-870.));
#37234=CARTESIAN_POINT('',(-8.19644660940673,9.54355339059324,-870.));
#37235=CARTESIAN_POINT('',(-11.5,6.24,-870.));
#37236=CARTESIAN_POINT('',(-8.05,9.89710678118652,-870.));
#37237=CARTESIAN_POINT('Origin',(-8.55,9.89710678118652,-870.));
#37238=CARTESIAN_POINT('',(-8.05,13.5928932188135,-870.));
#37239=CARTESIAN_POINT('',(-8.05,9.68999999999997,-870.));
#37240=CARTESIAN_POINT('',(-8.19644660940672,13.9464466094067,-870.));
#37241=CARTESIAN_POINT('Origin',(-8.55,13.5928932188135,-870.));
#37242=CARTESIAN_POINT('',(-8.57259699813414,14.3225969981341,-870.));
#37243=CARTESIAN_POINT('',(-8.05,13.8,-870.));
#37244=CARTESIAN_POINT('',(-8.71475010619428,14.6107663907404,-870.));
#37245=CARTESIAN_POINT('Origin',(-8.21904360754086,14.6761503887274,-870.));
#37246=CARTESIAN_POINT('',(-10.6942336092596,16.5902498938057,-870.));
#37247=CARTESIAN_POINT('Origin',(-10.995,14.31,-870.));
#37248=CARTESIAN_POINT('',(-10.9824030018658,16.7324030018659,-870.));
#37249=CARTESIAN_POINT('Origin',(-10.6288496112726,17.0859563924591,-870.));
#37250=CARTESIAN_POINT('',(-11.3535533905933,17.1035533905933,-870.));
#37251=CARTESIAN_POINT('',(-8.05,13.8,-870.));
#37252=CARTESIAN_POINT('',(-11.5,17.4571067811866,-870.));
#37253=CARTESIAN_POINT('Origin',(-11.,17.4571067811866,-870.));
#37254=CARTESIAN_POINT('',(-11.5,18.3428932188135,-870.));
#37255=CARTESIAN_POINT('',(-11.5,18.55,-870.));
#37256=CARTESIAN_POINT('',(-11.3535533905933,18.6964466094068,-870.));
#37257=CARTESIAN_POINT('Origin',(-11.,18.3428932188135,-870.));
#37258=CARTESIAN_POINT('',(-10.9824030018659,19.0675969981341,-870.));
#37259=CARTESIAN_POINT('',(-8.05,22.,-870.));
#37260=CARTESIAN_POINT('',(-10.6942336092596,19.2097501061943,-870.));
#37261=CARTESIAN_POINT('Origin',(-10.6288496112726,18.7140436075409,-870.));
#37262=CARTESIAN_POINT('',(-8.71475010619428,21.1892336092596,-870.));
#37263=CARTESIAN_POINT('Origin',(-10.995,21.49,-870.));
#37264=CARTESIAN_POINT('',(-8.57259699813413,21.4774030018659,-870.));
#37265=CARTESIAN_POINT('Origin',(-8.21904360754086,21.1238496112726,-870.));
#37266=CARTESIAN_POINT('',(-8.05,22.,-870.));
#37267=CARTESIAN_POINT('',(-8.05,22.,-870.));
#37268=CARTESIAN_POINT('',(8.05,22.,-870.));
#37269=CARTESIAN_POINT('',(-8.05,22.,-870.));
#37270=CARTESIAN_POINT('',(8.57259699813413,21.4774030018659,-870.));
#37271=CARTESIAN_POINT('',(8.05,22.,-870.));
#37272=CARTESIAN_POINT('',(8.71475010619428,21.1892336092596,-870.));
#37273=CARTESIAN_POINT('Origin',(8.21904360754086,21.1238496112726,-870.));
#37274=CARTESIAN_POINT('',(10.6942336092596,19.2097501061943,-870.));
#37275=CARTESIAN_POINT('Origin',(10.995,21.49,-870.));
#37276=CARTESIAN_POINT('',(10.9824030018659,19.0675969981341,-870.));
#37277=CARTESIAN_POINT('Origin',(10.6288496112726,18.7140436075409,-870.));
#37278=CARTESIAN_POINT('',(11.3535533905933,18.6964466094068,-870.));
#37279=CARTESIAN_POINT('',(8.05,22.,-870.));
#37280=CARTESIAN_POINT('',(11.5,18.3428932188135,-870.));
#37281=CARTESIAN_POINT('Origin',(11.,18.3428932188135,-870.));
#37282=CARTESIAN_POINT('',(11.5,17.4571067811866,-870.));
#37283=CARTESIAN_POINT('',(11.5,18.55,-870.));
#37284=CARTESIAN_POINT('',(11.3535533905933,17.1035533905933,-870.));
#37285=CARTESIAN_POINT('Origin',(11.,17.4571067811866,-870.));
#37286=CARTESIAN_POINT('',(10.9824030018658,16.7324030018659,-870.));
#37287=CARTESIAN_POINT('',(8.05,13.8,-870.));
#37288=CARTESIAN_POINT('',(10.6942336092596,16.5902498938057,-870.));
#37289=CARTESIAN_POINT('Origin',(10.6288496112726,17.0859563924591,-870.));
#37290=CARTESIAN_POINT('',(8.71475010619428,14.6107663907404,-870.));
#37291=CARTESIAN_POINT('Origin',(10.995,14.31,-870.));
#37292=CARTESIAN_POINT('',(8.57259699813414,14.3225969981341,-870.));
#37293=CARTESIAN_POINT('Origin',(8.21904360754086,14.6761503887274,-870.));
#37294=CARTESIAN_POINT('',(8.19644660940672,13.9464466094067,-870.));
#37295=CARTESIAN_POINT('',(8.05,13.8,-870.));
#37296=CARTESIAN_POINT('',(8.05,13.5928932188135,-870.));
#37297=CARTESIAN_POINT('Origin',(8.55,13.5928932188135,-870.));
#37298=CARTESIAN_POINT('',(8.05,9.89710678118651,-870.));
#37299=CARTESIAN_POINT('',(8.05,9.68999999999997,-870.));
#37300=CARTESIAN_POINT('',(8.19644660940673,9.54355339059324,-870.));
#37301=CARTESIAN_POINT('Origin',(8.55,9.89710678118651,-870.));
#37302=CARTESIAN_POINT('',(11.2071067811865,6.53289321881345,-870.));
#37303=CARTESIAN_POINT('',(11.5,6.24,-870.));
#37304=CARTESIAN_POINT('',(11.5,5.8257864376269,-870.));
#37305=CARTESIAN_POINT('Origin',(10.5,5.8257864376269,-870.));
#37306=CARTESIAN_POINT('',(11.5,1.00000000000001,-870.));
#37307=CARTESIAN_POINT('',(11.5,1.00000000000001,-870.));
#37308=CARTESIAN_POINT('',(10.5,-1.28587913910472E-15,-870.));
#37309=CARTESIAN_POINT('',(1.75,0.5,-870.));
#37310=CARTESIAN_POINT('',(1.75,0.5,-870.));
#37311=CARTESIAN_POINT('',(-1.75,0.5,-870.));
#37312=CARTESIAN_POINT('Origin',(0.,0.,30.));
#37313=CARTESIAN_POINT('',(-2.25,-1.4389599889981E-16,30.));
#37314=CARTESIAN_POINT('',(11.5,1.00000000000001,30.));
#37315=CARTESIAN_POINT('',(10.5,-1.28587913910472E-15,30.));
#37316=CARTESIAN_POINT('',(11.5,5.8257864376269,30.));
#37317=CARTESIAN_POINT('',(11.5,1.00000000000001,30.));
#37318=CARTESIAN_POINT('',(11.2071067811865,6.53289321881345,30.));
#37319=CARTESIAN_POINT('Origin',(10.5,5.8257864376269,30.));
#37320=CARTESIAN_POINT('',(8.19644660940673,9.54355339059324,30.));
#37321=CARTESIAN_POINT('',(11.5,6.24,30.));
#37322=CARTESIAN_POINT('',(8.05,9.89710678118651,30.));
#37323=CARTESIAN_POINT('Origin',(8.55,9.89710678118651,30.));
#37324=CARTESIAN_POINT('',(8.05,13.5928932188135,30.));
#37325=CARTESIAN_POINT('',(8.05,9.68999999999997,30.));
#37326=CARTESIAN_POINT('',(8.19644660940672,13.9464466094067,30.));
#37327=CARTESIAN_POINT('Origin',(8.55,13.5928932188135,30.));
#37328=CARTESIAN_POINT('',(8.57259699813414,14.3225969981341,30.));
#37329=CARTESIAN_POINT('',(8.05,13.8,30.));
#37330=CARTESIAN_POINT('',(8.71475010619428,14.6107663907404,30.));
#37331=CARTESIAN_POINT('Origin',(8.21904360754086,14.6761503887274,30.));
#37332=CARTESIAN_POINT('',(10.6942336092596,16.5902498938057,30.));
#37333=CARTESIAN_POINT('Origin',(10.995,14.31,30.));
#37334=CARTESIAN_POINT('',(10.9824030018658,16.7324030018659,30.));
#37335=CARTESIAN_POINT('Origin',(10.6288496112726,17.0859563924591,30.));
#37336=CARTESIAN_POINT('',(11.3535533905933,17.1035533905933,30.));
#37337=CARTESIAN_POINT('',(8.05,13.8,30.));
#37338=CARTESIAN_POINT('',(11.5,17.4571067811866,30.));
#37339=CARTESIAN_POINT('Origin',(11.,17.4571067811866,30.));
#37340=CARTESIAN_POINT('',(11.5,18.3428932188135,30.));
#37341=CARTESIAN_POINT('',(11.5,18.55,30.));
#37342=CARTESIAN_POINT('',(11.3535533905933,18.6964466094068,30.));
#37343=CARTESIAN_POINT('Origin',(11.,18.3428932188135,30.));
#37344=CARTESIAN_POINT('',(10.9824030018659,19.0675969981341,30.));
#37345=CARTESIAN_POINT('',(8.05,22.,30.));
#37346=CARTESIAN_POINT('',(10.6942336092596,19.2097501061943,30.));
#37347=CARTESIAN_POINT('Origin',(10.6288496112726,18.7140436075409,30.));
#37348=CARTESIAN_POINT('',(8.71475010619428,21.1892336092596,30.));
#37349=CARTESIAN_POINT('Origin',(10.995,21.49,30.));
#37350=CARTESIAN_POINT('',(8.57259699813413,21.4774030018659,30.));
#37351=CARTESIAN_POINT('Origin',(8.21904360754086,21.1238496112726,30.));
#37352=CARTESIAN_POINT('',(8.05,22.,30.));
#37353=CARTESIAN_POINT('',(8.05,22.,30.));
#37354=CARTESIAN_POINT('',(-8.05,22.,30.));
#37355=CARTESIAN_POINT('',(-8.05,22.,30.));
#37356=CARTESIAN_POINT('',(-8.57259699813413,21.4774030018659,30.));
#37357=CARTESIAN_POINT('',(-8.05,22.,30.));
#37358=CARTESIAN_POINT('',(-8.71475010619428,21.1892336092596,30.));
#37359=CARTESIAN_POINT('Origin',(-8.21904360754086,21.1238496112726,30.));
#37360=CARTESIAN_POINT('',(-10.6942336092596,19.2097501061943,30.));
#37361=CARTESIAN_POINT('Origin',(-10.995,21.49,30.));
#37362=CARTESIAN_POINT('',(-10.9824030018659,19.0675969981341,30.));
#37363=CARTESIAN_POINT('Origin',(-10.6288496112726,18.7140436075409,30.));
#37364=CARTESIAN_POINT('',(-11.3535533905933,18.6964466094068,30.));
#37365=CARTESIAN_POINT('',(-8.05,22.,30.));
#37366=CARTESIAN_POINT('',(-11.5,18.3428932188135,30.));
#37367=CARTESIAN_POINT('Origin',(-11.,18.3428932188135,30.));
#37368=CARTESIAN_POINT('',(-11.5,17.4571067811866,30.));
#37369=CARTESIAN_POINT('',(-11.5,18.55,30.));
#37370=CARTESIAN_POINT('',(-11.3535533905933,17.1035533905933,30.));
#37371=CARTESIAN_POINT('Origin',(-11.,17.4571067811866,30.));
#37372=CARTESIAN_POINT('',(-10.9824030018658,16.7324030018659,30.));
#37373=CARTESIAN_POINT('',(-8.05,13.8,30.));
#37374=CARTESIAN_POINT('',(-10.6942336092596,16.5902498938057,30.));
#37375=CARTESIAN_POINT('Origin',(-10.6288496112726,17.0859563924591,30.));
#37376=CARTESIAN_POINT('',(-8.71475010619428,14.6107663907404,30.));
#37377=CARTESIAN_POINT('Origin',(-10.995,14.31,30.));
#37378=CARTESIAN_POINT('',(-8.57259699813414,14.3225969981341,30.));
#37379=CARTESIAN_POINT('Origin',(-8.21904360754086,14.6761503887274,30.));
#37380=CARTESIAN_POINT('',(-8.19644660940672,13.9464466094067,30.));
#37381=CARTESIAN_POINT('',(-8.05,13.8,30.));
#37382=CARTESIAN_POINT('',(-8.05,13.5928932188135,30.));
#37383=CARTESIAN_POINT('Origin',(-8.55,13.5928932188135,30.));
#37384=CARTESIAN_POINT('',(-8.05,9.89710678118652,30.));
#37385=CARTESIAN_POINT('',(-8.05,9.68999999999997,30.));
#37386=CARTESIAN_POINT('',(-8.19644660940673,9.54355339059324,30.));
#37387=CARTESIAN_POINT('Origin',(-8.55,9.89710678118652,30.));
#37388=CARTESIAN_POINT('',(-11.2071067811865,6.53289321881345,30.));
#37389=CARTESIAN_POINT('',(-11.5,6.24,30.));
#37390=CARTESIAN_POINT('',(-11.5,5.8257864376269,30.));
#37391=CARTESIAN_POINT('Origin',(-10.5,5.8257864376269,30.));
#37392=CARTESIAN_POINT('',(-11.5,1.00000000000001,30.));
#37393=CARTESIAN_POINT('',(-11.5,1.00000000000001,30.));
#37394=CARTESIAN_POINT('',(-10.5,-1.28587913910472E-15,30.));
#37395=CARTESIAN_POINT('Origin',(8.05,13.8,-870.));
#37396=CARTESIAN_POINT('',(8.19644660940672,13.9464466094067,-870.));
#37397=CARTESIAN_POINT('',(8.57259699813414,14.3225969981341,30.));
#37398=CARTESIAN_POINT('Origin',(8.05,13.8,-870.));
#37399=CARTESIAN_POINT('',(11.3535533905933,17.1035533905933,-870.));
#37400=CARTESIAN_POINT('',(10.9824030018658,16.7324030018659,-870.));
#37401=CARTESIAN_POINT('Origin',(8.05,22.,-870.));
#37402=CARTESIAN_POINT('',(10.9824030018659,19.0675969981341,30.));
#37403=CARTESIAN_POINT('',(11.3535533905933,18.6964466094068,-870.));
#37404=CARTESIAN_POINT('Origin',(8.05,22.,-870.));
#37405=CARTESIAN_POINT('',(8.57259699813413,21.4774030018659,-870.));
#37406=CARTESIAN_POINT('',(8.05,22.,-870.));
#37407=CARTESIAN_POINT('Origin',(-8.05,13.8,-870.));
#37408=CARTESIAN_POINT('',(-8.19644660940672,13.9464466094067,30.));
#37409=CARTESIAN_POINT('',(-8.57259699813414,14.3225969981341,-870.));
#37410=CARTESIAN_POINT('Origin',(-8.05,22.,-870.));
#37411=CARTESIAN_POINT('',(-10.9824030018659,19.0675969981341,-870.));
#37412=CARTESIAN_POINT('',(-11.3535533905933,18.6964466094068,-870.));
#37413=CARTESIAN_POINT('Origin',(-8.05,22.,-870.));
#37414=CARTESIAN_POINT('',(-8.05,22.,-870.));
#37415=CARTESIAN_POINT('Origin',(-10.5,-1.28587913910472E-15,-870.));
#37416=CARTESIAN_POINT('',(-11.5,1.00000000000001,-870.));
#37417=CARTESIAN_POINT('Origin',(-11.5,1.00000000000001,-870.));
#37418=CARTESIAN_POINT('',(-11.5,5.8257864376269,-870.));
#37419=CARTESIAN_POINT('Origin',(-11.5,6.24,-870.));
#37420=CARTESIAN_POINT('',(-11.2071067811865,6.53289321881345,-870.));
#37421=CARTESIAN_POINT('',(-8.19644660940673,9.54355339059324,-870.));
#37422=CARTESIAN_POINT('Origin',(-8.05,9.68999999999997,-870.));
#37423=CARTESIAN_POINT('',(-8.05,9.89710678118652,30.));
#37424=CARTESIAN_POINT('',(-8.05,13.5928932188135,-870.));
#37425=CARTESIAN_POINT('Origin',(-8.05,13.8,-870.));
#37426=CARTESIAN_POINT('',(-11.3535533905933,17.1035533905933,-870.));
#37427=CARTESIAN_POINT('',(-10.9824030018658,16.7324030018659,30.));
#37428=CARTESIAN_POINT('Origin',(-11.5,18.55,-870.));
#37429=CARTESIAN_POINT('',(-11.5,18.3428932188135,-870.));
#37430=CARTESIAN_POINT('',(-11.5,17.4571067811866,-870.));
#37431=CARTESIAN_POINT('Origin',(-8.05,22.,-870.));
#37432=CARTESIAN_POINT('',(-8.57259699813413,21.4774030018659,30.));
#37433=CARTESIAN_POINT('Origin',(-10.995,21.49,-870.));
#37434=CARTESIAN_POINT('',(-10.6942336092596,19.2097501061943,-870.));
#37435=CARTESIAN_POINT('',(-8.71475010619428,21.1892336092596,-870.));
#37436=CARTESIAN_POINT('Origin',(-10.995,14.31,-870.));
#37437=CARTESIAN_POINT('',(-10.6942336092596,16.5902498938057,-870.));
#37438=CARTESIAN_POINT('',(-8.71475010619428,14.6107663907404,-870.));
#37439=CARTESIAN_POINT('Origin',(-10.6288496112726,18.7140436075409,-870.));
#37440=CARTESIAN_POINT('Origin',(-11.,18.3428932188135,-870.));
#37441=CARTESIAN_POINT('Origin',(-11.,17.4571067811866,-870.));
#37442=CARTESIAN_POINT('Origin',(-10.6288496112726,17.0859563924591,-870.));
#37443=CARTESIAN_POINT('Origin',(-8.55,9.89710678118652,-870.));
#37444=CARTESIAN_POINT('Origin',(-8.55,13.5928932188135,-870.));
#37445=CARTESIAN_POINT('Origin',(-8.21904360754086,14.6761503887274,-870.));
#37446=CARTESIAN_POINT('Origin',(-8.21904360754086,21.1238496112726,-870.));
#37447=CARTESIAN_POINT('Origin',(-10.5,5.8257864376269,-870.));
#37448=CARTESIAN_POINT('Origin',(11.5,18.55,-870.));
#37449=CARTESIAN_POINT('',(11.5,18.3428932188135,-870.));
#37450=CARTESIAN_POINT('',(11.5,17.4571067811866,-870.));
#37451=CARTESIAN_POINT('Origin',(8.05,9.68999999999997,-870.));
#37452=CARTESIAN_POINT('',(8.05,9.89710678118651,-870.));
#37453=CARTESIAN_POINT('',(8.05,13.5928932188135,30.));
#37454=CARTESIAN_POINT('Origin',(11.5,6.24,-870.));
#37455=CARTESIAN_POINT('',(11.2071067811865,6.53289321881345,-870.));
#37456=CARTESIAN_POINT('',(8.19644660940673,9.54355339059324,30.));
#37457=CARTESIAN_POINT('Origin',(11.5,1.00000000000001,-870.));
#37458=CARTESIAN_POINT('',(11.5,5.8257864376269,-870.));
#37459=CARTESIAN_POINT('',(11.5,1.00000000000001,-870.));
#37460=CARTESIAN_POINT('Origin',(10.5,-1.28587913910472E-15,-870.));
#37461=CARTESIAN_POINT('Origin',(10.995,21.49,-870.));
#37462=CARTESIAN_POINT('',(10.6942336092596,19.2097501061943,-870.));
#37463=CARTESIAN_POINT('',(8.71475010619428,21.1892336092596,-870.));
#37464=CARTESIAN_POINT('Origin',(10.995,14.31,-870.));
#37465=CARTESIAN_POINT('',(10.6942336092596,16.5902498938057,-870.));
#37466=CARTESIAN_POINT('',(8.71475010619428,14.6107663907404,-870.));
#37467=CARTESIAN_POINT('Origin',(10.6288496112726,18.7140436075409,-870.));
#37468=CARTESIAN_POINT('Origin',(11.,18.3428932188135,-870.));
#37469=CARTESIAN_POINT('Origin',(11.,17.4571067811866,-870.));
#37470=CARTESIAN_POINT('Origin',(10.6288496112726,17.0859563924591,-870.));
#37471=CARTESIAN_POINT('Origin',(8.55,9.89710678118651,-870.));
#37472=CARTESIAN_POINT('Origin',(8.55,13.5928932188135,-870.));
#37473=CARTESIAN_POINT('Origin',(8.21904360754086,14.6761503887274,-870.));
#37474=CARTESIAN_POINT('Origin',(8.21904360754086,21.1238496112726,-870.));
#37475=CARTESIAN_POINT('Origin',(10.5,5.8257864376269,-870.));
#37476=CARTESIAN_POINT('Origin',(-2.25,-1.4389599889981E-16,-870.));
#37477=CARTESIAN_POINT('Origin',(-1.75,0.5,-870.));
#37478=CARTESIAN_POINT('',(1.75,0.5,-870.));
#37479=CARTESIAN_POINT('Origin',(1.75,0.5,-870.));
#37480=CARTESIAN_POINT('Origin',(3.5,13.,0.));
#37481=CARTESIAN_POINT('Origin',(3.5,13.,-60.));
#37482=CARTESIAN_POINT('Origin',(3.5,13.,-120.));
#37483=CARTESIAN_POINT('Origin',(3.5,13.,-180.));
#37484=CARTESIAN_POINT('Origin',(3.5,13.,-240.));
#37485=CARTESIAN_POINT('Origin',(3.5,13.,-300.));
#37486=CARTESIAN_POINT('Origin',(3.5,13.,-360.));
#37487=CARTESIAN_POINT('Origin',(3.5,13.,-420.));
#37488=CARTESIAN_POINT('Origin',(3.5,13.,-480.));
#37489=CARTESIAN_POINT('Origin',(3.5,13.,-540.));
#37490=CARTESIAN_POINT('Origin',(3.5,13.,-600.));
#37491=CARTESIAN_POINT('Origin',(3.5,13.,-660.));
#37492=CARTESIAN_POINT('Origin',(3.5,13.,-720.));
#37493=CARTESIAN_POINT('Origin',(3.5,13.,-780.));
#37494=CARTESIAN_POINT('Origin',(3.5,13.,-840.));
#66650=UNCERTAINTY_MEASURE_WITH_UNIT(LENGTH_MEASURE(0.01),#66722,
'DISTANCE_ACCURACY_VALUE',
'Maximum model space distance between geometric entities at asserted c
onnectivities');
#66680=UNCERTAINTY_MEASURE_WITH_UNIT(LENGTH_MEASURE(0.01),#66722,
'DISTANCE_ACCURACY_VALUE',
'Maximum model space distance between geometric entities at asserted c
onnectivities');
#66691=(
GEOMETRIC_REPRESENTATION_CONTEXT(3)
GLOBAL_UNCERTAINTY_ASSIGNED_CONTEXT((#66650))
GLOBAL_UNIT_ASSIGNED_CONTEXT((#66722,#66724,#66725))
REPRESENTATION_CONTEXT('','3D')
);
#66721=(
GEOMETRIC_REPRESENTATION_CONTEXT(3)
GLOBAL_UNCERTAINTY_ASSIGNED_CONTEXT((#66680))
GLOBAL_UNIT_ASSIGNED_CONTEXT((#66722,#66724,#66725))
REPRESENTATION_CONTEXT('','3D')
);
#66722=(
LENGTH_UNIT()
NAMED_UNIT(*)
SI_UNIT(.MILLI.,.METRE.)
);
#66724=(
NAMED_UNIT(*)
PLANE_ANGLE_UNIT()
SI_UNIT($,.RADIAN.)
);
#66725=(
NAMED_UNIT(*)
SI_UNIT($,.STERADIAN.)
SOLID_ANGLE_UNIT()
);
#66736=SHAPE_DEFINITION_REPRESENTATION(#66778,#66900);
#66778=PRODUCT_DEFINITION_SHAPE('',$,#66941);
#66900=SHAPE_REPRESENTATION('',(#26229),#66691);
#66930=PRODUCT_DEFINITION_CONTEXT('part definition',#67052,'design');
#66941=PRODUCT_DEFINITION('Linear Guide Rail','Linear Guide Rail',#66981,
#66930);
#66981=PRODUCT_DEFINITION_FORMATION('',$,#67064);
#67052=APPLICATION_CONTEXT(
'Core Data for Automotive Mechanical Design Process');
#67053=PRODUCT_CONTEXT('part definition',#67052,'mechanical');
#67064=PRODUCT('Linear Guide Rail','Linear Guide Rail',$,(#67053));
#67095=PRESENTATION_STYLE_ASSIGNMENT((#67097));
#67097=SURFACE_STYLE_USAGE(.BOTH.,#67099);
#67099=SURFACE_SIDE_STYLE('',(#67101));
#67101=SURFACE_STYLE_FILL_AREA(#67103);
#67103=FILL_AREA_STYLE('Opaque(202,209,238)',(#67105));
#67105=FILL_AREA_STYLE_COLOUR('Opaque(202,209,238)',#67107);
#67107=COLOUR_RGB('Opaque(202,209,238)',0.792156862745098,0.819607843137255,
0.933333333333333);
ENDSEC;
END-ISO-10303-21;
